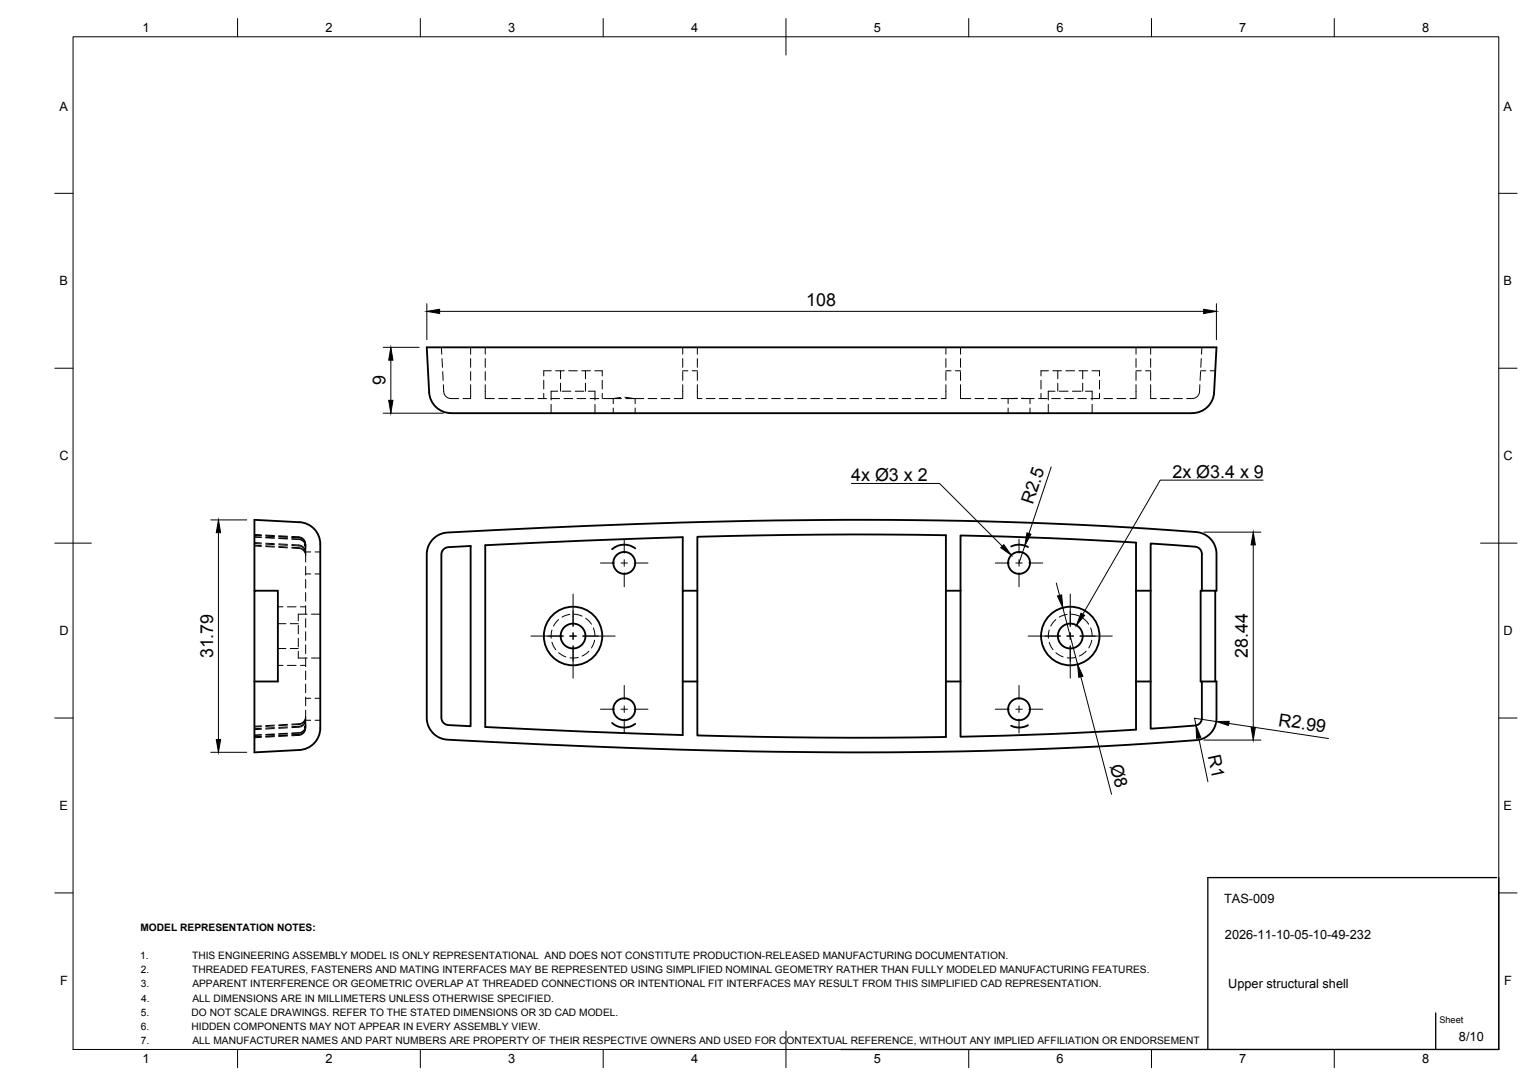
ISO-10303-21;
HEADER;
/* Generated by software containing ST-Developer
 * from STEP Tools, Inc. (www.steptools.com) 
 */

FILE_DESCRIPTION(
/* description */ (''),
/* implementation_level */ '2;1');

FILE_NAME(
/* name */ 'Upper structural shell.step',
/* time_stamp */ '2026-11-12T00:53:40-08:00',
/* author */ (''),
/* organization */ (''),
/* preprocessor_version */ 'ST-DEVELOPER v20.2',
/* originating_system */ 'Autodesk Translation Framework v15.17.0.0',
/* authorisation */ '');

FILE_SCHEMA (('AUTOMOTIVE_DESIGN { 1 0 10303 214 3 1 1 }'));
ENDSEC;

DATA;
#10=MECHANICAL_DESIGN_GEOMETRIC_PRESENTATION_REPRESENTATION('',(#575),#22129);
#76=SPHERICAL_SURFACE('',#9161,0.1);
#77=SPHERICAL_SURFACE('',#9164,0.0999999999999998);
#78=SPHERICAL_SURFACE('',#9168,0.0999999999999993);
#79=SPHERICAL_SURFACE('',#9172,0.1);
#80=SPHERICAL_SURFACE('',#9177,0.3);
#81=SPHERICAL_SURFACE('',#9181,0.3);
#82=SPHERICAL_SURFACE('',#9185,0.299999999999999);
#83=SPHERICAL_SURFACE('',#9190,0.3);
#92=B_SPLINE_SURFACE_WITH_KNOTS('',3,3,((#12365,#12366,#12367,#12368),(#12369,
#12370,#12371,#12372),(#12373,#12374,#12375,#12376),(#12377,#12378,#12379,
#12380),(#12381,#12382,#12383,#12384)),.UNSPECIFIED.,.F.,.F.,.F.,(4,1,4),
(4,4),(0.,0.571428571428571,1.),(1.0454440030657,3.44967454744645),
 .UNSPECIFIED.);
#93=B_SPLINE_SURFACE_WITH_KNOTS('',3,3,((#12457,#12458,#12459,#12460),(#12461,
#12462,#12463,#12464),(#12465,#12466,#12467,#12468),(#12469,#12470,#12471,
#12472),(#12473,#12474,#12475,#12476)),.UNSPECIFIED.,.F.,.F.,.F.,(4,1,4),
(4,4),(0.,0.571428571428571,1.),(7.24519303641511,9.95046872158573),
 .UNSPECIFIED.);
#94=B_SPLINE_SURFACE_WITH_KNOTS('',3,3,((#13338,#13339,#13340,#13341),(#13342,
#13343,#13344,#13345),(#13346,#13347,#13348,#13349),(#13350,#13351,#13352,
#13353)),.UNSPECIFIED.,.F.,.F.,.F.,(4,4),(4,4),(0.0705535719740953,0.323522444336189),
(0.0117434863834119,0.684857763552191),.UNSPECIFIED.);
#95=B_SPLINE_SURFACE_WITH_KNOTS('',3,3,((#13358,#13359,#13360,#13361),(#13362,
#13363,#13364,#13365),(#13366,#13367,#13368,#13369),(#13370,#13371,#13372,
#13373)),.UNSPECIFIED.,.F.,.F.,.F.,(4,4),(4,4),(0.0262419052680539,0.0545428296147404),
(0.0121538053864343,0.684980602226481),.UNSPECIFIED.);
#96=B_SPLINE_SURFACE_WITH_KNOTS('',3,3,((#13383,#13384,#13385,#13386),(#13387,
#13388,#13389,#13390),(#13391,#13392,#13393,#13394),(#13395,#13396,#13397,
#13398),(#13399,#13400,#13401,#13402)),.UNSPECIFIED.,.F.,.F.,.F.,(4,1,4),
(4,4),(0.,0.571428571428571,1.),(0.752061768057538,3.45733745322815),
 .UNSPECIFIED.);
#97=B_SPLINE_SURFACE_WITH_KNOTS('',3,3,((#13403,#13404,#13405,#13406),(#13407,
#13408,#13409,#13410),(#13411,#13412,#13413,#13414),(#13415,#13416,#13417,
#13418),(#13419,#13420,#13421,#13422)),.UNSPECIFIED.,.F.,.F.,.F.,(4,1,4),
(4,4),(0.,0.571428571428571,1.),(0.283259008618247,0.557056952888827),
 .UNSPECIFIED.);
#98=B_SPLINE_SURFACE_WITH_KNOTS('',3,3,((#13436,#13437,#13438,#13439),(#13440,
#13441,#13442,#13443),(#13444,#13445,#13446,#13447),(#13448,#13449,#13450,
#13451)),.UNSPECIFIED.,.F.,.F.,.F.,(4,4),(4,4),(0.67647755566375,0.929446428026011),
(0.0117434863436937,0.684857763580381),.UNSPECIFIED.);
#99=B_SPLINE_SURFACE_WITH_KNOTS('',3,3,((#13452,#13453,#13454,#13455),(#13456,
#13457,#13458,#13459),(#13460,#13461,#13462,#13463),(#13464,#13465,#13466,
#13467)),.UNSPECIFIED.,.F.,.F.,.F.,(4,4),(4,4),(0.945457170385156,0.973758094731946),
(0.0121538053598088,0.684980602226481),.UNSPECIFIED.);
#100=B_SPLINE_SURFACE_WITH_KNOTS('',3,3,((#13551,#13552,#13553,#13554),
(#13555,#13556,#13557,#13558),(#13559,#13560,#13561,#13562),(#13563,#13564,
#13565,#13566)),.UNSPECIFIED.,.F.,.F.,.F.,(4,4),(4,4),(0.341142793678372,
0.658675488550287),(0.0116221239297273,0.684255166525269),.UNSPECIFIED.);
#101=B_SPLINE_SURFACE_WITH_KNOTS('',3,3,((#13571,#13572,#13573,#13574),
(#13575,#13576,#13577,#13578),(#13579,#13580,#13581,#13582),(#13583,#13584,
#13585,#13586),(#13587,#13588,#13589,#13590)),.UNSPECIFIED.,.F.,.F.,.F.,
(4,1,4),(4,4),(0.,0.571428571428571,1.),(3.65450559744172,7.0548588409572),
 .UNSPECIFIED.);
#102=B_SPLINE_SURFACE_WITH_KNOTS('',3,3,((#13600,#13601,#13602,#13603),
(#13604,#13605,#13606,#13607),(#13608,#13609,#13610,#13611),(#13612,#13613,
#13614,#13615),(#13616,#13617,#13618,#13619)),.UNSPECIFIED.,.F.,.F.,.F.,
(4,1,4),(4,4),(0.,0.571428571428571,1.),(3.64767164868607,7.04802489220155),
 .UNSPECIFIED.);
#103=B_SPLINE_SURFACE_WITH_KNOTS('',3,3,((#13624,#13625,#13626,#13627),
(#13628,#13629,#13630,#13631),(#13632,#13633,#13634,#13635),(#13636,#13637,
#13638,#13639)),.UNSPECIFIED.,.F.,.F.,.F.,(4,4),(4,4),(0.341324511449716,
0.658857206321627),(0.0116221214776208,0.684255166525269),.UNSPECIFIED.);
#104=B_SPLINE_SURFACE_WITH_KNOTS('',3,3,((#13684,#13685,#13686,#13687),
(#13688,#13689,#13690,#13691),(#13692,#13693,#13694,#13695),(#13696,#13697,
#13698,#13699)),.UNSPECIFIED.,.F.,.F.,.F.,(4,4),(4,4),(0.676316266718331,
0.901708040522105),(0.0117102006467275,0.68495201331719),.UNSPECIFIED.);
#105=B_SPLINE_SURFACE_WITH_KNOTS('',3,3,((#13704,#13705,#13706,#13707),
(#13708,#13709,#13710,#13711),(#13712,#13713,#13714,#13715),(#13716,#13717,
#13718,#13719),(#13720,#13721,#13722,#13723)),.UNSPECIFIED.,.F.,.F.,.F.,
(4,1,4),(4,4),(0.,0.571428571428571,1.),(7.25285594219682,9.65708648657758),
 .UNSPECIFIED.);
#106=B_SPLINE_SURFACE_WITH_KNOTS('',3,3,((#13733,#13734,#13735,#13736),
(#13737,#13738,#13739,#13740),(#13741,#13742,#13743,#13744),(#13745,#13746,
#13747,#13748)),.UNSPECIFIED.,.F.,.F.,.F.,(4,4),(4,4),(0.0982919594778951,
0.323683733281714),(0.0117102006467272,0.68495201331719),.UNSPECIFIED.);
#107=B_SPLINE_SURFACE_WITH_KNOTS('',3,3,((#13823,#13824,#13825,#13826),
(#13827,#13828,#13829,#13830),(#13831,#13832,#13833,#13834),(#13835,#13836,
#13837,#13838)),.UNSPECIFIED.,.F.,.F.,.F.,(4,4),(4,4),(0.917922863855343,
0.974411608827007),(0.0122403473423911,0.685344304754238),.UNSPECIFIED.);
#108=B_SPLINE_SURFACE_WITH_KNOTS('',3,3,((#13848,#13849,#13850,#13851),
(#13852,#13853,#13854,#13855),(#13856,#13857,#13858,#13859),(#13860,#13861,
#13862,#13863),(#13864,#13865,#13866,#13867)),.UNSPECIFIED.,.F.,.F.,.F.,
(4,1,4),(4,4),(0.,0.571428571428571,1.),(9.85085636625011,10.4271318523291),
 .UNSPECIFIED.);
#109=B_SPLINE_SURFACE_WITH_KNOTS('',3,3,((#13881,#13882,#13883,#13884),
(#13885,#13886,#13887,#13888),(#13889,#13890,#13891,#13892),(#13893,#13894,
#13895,#13896)),.UNSPECIFIED.,.F.,.F.,.F.,(4,4),(4,4),(0.025588391172993,
0.0820771361446569),(0.0122403473423911,0.685344304754238),
 .UNSPECIFIED.);
#110=B_SPLINE_SURFACE_WITH_KNOTS('',3,3,((#13906,#13907,#13908,#13909),
(#13910,#13911,#13912,#13913),(#13914,#13915,#13916,#13917),(#13918,#13919,
#13920,#13921),(#13922,#13923,#13924,#13925)),.UNSPECIFIED.,.F.,.F.,.F.,
(4,1,4),(4,4),(0.,0.571428571428571,1.),(0.27539863731415,0.851674123393175),
 .UNSPECIFIED.);
#111=B_SPLINE_SURFACE_WITH_KNOTS('',3,3,((#13939,#13940,#13941,#13942),
(#13943,#13944,#13945,#13946),(#13947,#13948,#13949,#13950),(#13951,#13952,
#13953,#13954),(#13955,#13956,#13957,#13958)),.UNSPECIFIED.,.F.,.F.,.F.,
(4,1,4),(4,4),(0.,0.571428571428571,1.),(0.00944995813270487,0.618489359031386),
 .UNSPECIFIED.);
#112=B_SPLINE_SURFACE_WITH_KNOTS('',3,3,((#13965,#13966,#13967,#13968),
(#13969,#13970,#13971,#13972),(#13973,#13974,#13975,#13976),(#13977,#13978,
#13979,#13980),(#13981,#13982,#13983,#13984)),.UNSPECIFIED.,.F.,.F.,.F.,
(4,1,4),(4,4),(0.,0.571428571428571,1.),(0.00908570715245136,0.618164468641375),
 .UNSPECIFIED.);
#113=B_SPLINE_SURFACE_WITH_KNOTS('',3,3,((#13989,#13990,#13991,#13992),
(#13993,#13994,#13995,#13996),(#13997,#13998,#13999,#14000),(#14001,#14002,
#14003,#14004),(#14005,#14006,#14007,#14008)),.UNSPECIFIED.,.F.,.F.,.F.,
(4,1,4),(4,4),(0.,0.571428571428571,1.),(0.0091183540525243,0.618164468641375),
 .UNSPECIFIED.);
#114=B_SPLINE_SURFACE_WITH_KNOTS('',3,3,((#14013,#14014,#14015,#14016),
(#14017,#14018,#14019,#14020),(#14021,#14022,#14023,#14024),(#14025,#14026,
#14027,#14028),(#14029,#14030,#14031,#14032)),.UNSPECIFIED.,.F.,.F.,.F.,
(4,1,4),(4,4),(0.,0.571428571428571,1.),(10.1454735367545,10.419271481025),
 .UNSPECIFIED.);
#115=B_SPLINE_SURFACE_WITH_KNOTS('',3,3,((#14033,#14034,#14035,#14036),
(#14037,#14038,#14039,#14040),(#14041,#14042,#14043,#14044),(#14045,#14046,
#14047,#14048),(#14049,#14050,#14051,#14052)),.UNSPECIFIED.,.F.,.F.,.F.,
(4,1,4),(4,4),(0.,0.571428571428571,1.),(0.0094045468285345,0.618489359031386),
 .UNSPECIFIED.);
#116=B_SPLINE_SURFACE_WITH_KNOTS('',3,3,((#14078,#14079,#14080,#14081),
(#14082,#14083,#14084,#14085),(#14086,#14087,#14088,#14089),(#14090,#14091,
#14092,#14093),(#14094,#14095,#14096,#14097)),.UNSPECIFIED.,.F.,.F.,.F.,
(4,1,4),(4,4),(0.,0.571428571428571,1.),(-0.00535061636073277,0.618489359031386),
 .UNSPECIFIED.);
#117=B_SPLINE_SURFACE_WITH_KNOTS('',3,3,((#14116,#14117,#14118,#14119,#14120),
(#14121,#14122,#14123,#14124,#14125),(#14126,#14127,#14128,#14129,#14130),
(#14131,#14132,#14133,#14134,#14135),(#14136,#14137,#14138,#14139,#14140)),
 .UNSPECIFIED.,.F.,.F.,.F.,(4,1,4),(4,1,4),(0.,0.571428571428571,1.),(0.283259008618247,
4.63063308449434,10.4271318523291),.UNSPECIFIED.);
#118=B_SPLINE_SURFACE_WITH_KNOTS('',3,3,((#14151,#14152,#14153,#14154),
(#14155,#14156,#14157,#14158),(#14159,#14160,#14161,#14162),(#14163,#14164,
#14165,#14166),(#14167,#14168,#14169,#14170)),.UNSPECIFIED.,.F.,.F.,.F.,
(4,1,4),(4,4),(0.,0.571428571428571,1.),(-0.00578978989683084,0.618164468641375),
 .UNSPECIFIED.);
#119=B_SPLINE_SURFACE_WITH_KNOTS('',3,3,((#14179,#14180,#14181,#14182),
(#14183,#14184,#14185,#14186),(#14187,#14188,#14189,#14190),(#14191,#14192,
#14193,#14194),(#14195,#14196,#14197,#14198)),.UNSPECIFIED.,.F.,.F.,.F.,
(4,1,4),(4,4),(0.,0.571428571428571,1.),(-0.00569189159989896,0.618164468641375),
 .UNSPECIFIED.);
#120=B_SPLINE_SURFACE_WITH_KNOTS('',3,3,((#14207,#14208,#14209,#14210,#14211),
(#14212,#14213,#14214,#14215,#14216),(#14217,#14218,#14219,#14220,#14221),
(#14222,#14223,#14224,#14225,#14226),(#14227,#14228,#14229,#14230,#14231)),
 .UNSPECIFIED.,.F.,.F.,.F.,(4,1,4),(4,1,4),(0.,0.571428571428571,1.),(0.27539863731415,
4.62277271319024,10.419271481025),.UNSPECIFIED.);
#121=B_SPLINE_SURFACE_WITH_KNOTS('',3,3,((#14242,#14243,#14244,#14245),
(#14246,#14247,#14248,#14249),(#14250,#14251,#14252,#14253),(#14254,#14255,
#14256,#14257),(#14258,#14259,#14260,#14261)),.UNSPECIFIED.,.F.,.F.,.F.,
(4,1,4),(4,4),(0.,0.571428571428571,1.),(-0.0054868135546625,0.618489359031386),
 .UNSPECIFIED.);
#122=B_SPLINE_SURFACE_WITH_KNOTS('',3,3,((#14270,#14271,#14272,#14273),
(#14274,#14275,#14276,#14277),(#14278,#14279,#14280,#14281),(#14282,#14283,
#14284,#14285)),.UNSPECIFIED.,.F.,.F.,.F.,(4,4),(4,4),(0.026239262514127,
0.974414173651419),(0.,0.685344304754238),.UNSPECIFIED.);
#123=B_SPLINE_SURFACE_WITH_KNOTS('',3,3,((#14288,#14289,#14290,#14291),
(#14292,#14293,#14294,#14295),(#14296,#14297,#14298,#14299),(#14300,#14301,
#14302,#14303)),.UNSPECIFIED.,.F.,.F.,.F.,(4,4),(4,4),(0.0255858263485814,
0.973760737485873),(0.,0.685344304754238),.UNSPECIFIED.);
#172=B_SPLINE_CURVE_WITH_KNOTS('',3,(#12264,#12265,#12266,#12267,#12268,
#12269,#12270,#12271,#12272,#12273,#12274,#12275,#12276,#12277,#12278,#12279,
#12280,#12281,#12282,#12283,#12284,#12285,#12286,#12287),.UNSPECIFIED.,
 .F.,.F.,(4,2,2,2,2,2,2,2,2,2,2,4),(-0.337265338267783,-0.250544943628509,
-0.208272806508042,-0.186542211788094,-0.176382978682897,-0.170925844043069,
-0.16639450677335,-0.161077381235501,-0.15182241135393,-0.115009181549223,
-0.030206004227969,0.),.UNSPECIFIED.);
#173=B_SPLINE_CURVE_WITH_KNOTS('',3,(#12292,#12293,#12294,#12295,#12296,
#12297,#12298,#12299,#12300,#12301,#12302,#12303,#12304,#12305,#12306,#12307,
#12308,#12309,#12310,#12311),.UNSPECIFIED.,.F.,.F.,(4,2,2,2,2,2,2,2,2,4),
(-0.240982594686416,-0.16829976149504,-0.141836598208813,-0.129116059226128,
-0.121962912034391,-0.115857591426886,-0.108506552485159,-0.0948769875819265,
-0.0364654790774683,0.),.UNSPECIFIED.);
#174=B_SPLINE_CURVE_WITH_KNOTS('',3,(#12316,#12317,#12318,#12319,#12320,
#12321,#12322,#12323,#12324,#12325,#12326,#12327,#12328,#12329,#12330,#12331,
#12332,#12333,#12334,#12335),.UNSPECIFIED.,.F.,.F.,(4,2,2,2,2,2,2,2,2,4),
(-0.240981214998207,-0.168303541671295,-0.141841407502325,-0.129121097580905,
-0.121968013294536,-0.115862708924237,-0.108511643765797,-0.0948818976588229,
-0.0364681276985956,0.),.UNSPECIFIED.);
#175=B_SPLINE_CURVE_WITH_KNOTS('',3,(#12340,#12341,#12342,#12343,#12344,
#12345,#12346,#12347,#12348,#12349,#12350,#12351,#12352,#12353,#12354,#12355,
#12356,#12357,#12358,#12359,#12360,#12361,#12362,#12363),.UNSPECIFIED.,
 .F.,.F.,(4,2,2,2,2,2,2,2,2,2,2,4),(-0.337269388373684,-0.250545316912909,
-0.208282401844766,-0.186554569827561,-0.176396213396297,-0.17093921790305,
-0.16640782243471,-0.161090427650893,-0.151834477986603,-0.115010808423941,
-0.0302102096065556,0.),.UNSPECIFIED.);
#176=B_SPLINE_CURVE_WITH_KNOTS('',3,(#12386,#12387,#12388,#12389),
 .UNSPECIFIED.,.F.,.F.,(4,4),(1.0454440030657,2.52465537163019),
 .UNSPECIFIED.);
#177=B_SPLINE_CURVE_WITH_KNOTS('',3,(#12391,#12392,#12393,#12394,#12395,
#12396,#12397,#12398,#12399,#12400,#12401,#12402,#12403,#12404,#12405,#12406,
#12407,#12408,#12409,#12410,#12411,#12412,#12413,#12414,#12415,#12416,#12417,
#12418),.UNSPECIFIED.,.F.,.F.,(4,3,3,3,3,3,3,3,3,4),(-0.152193408756968,
-0.128427023368412,-0.115107736263918,-0.0911810900745799,-0.0780377802127556,
-0.0652031397886901,-0.0414031558437525,-0.0389949527774582,-0.0152076153333754,
0.),.UNSPECIFIED.);
#178=B_SPLINE_CURVE_WITH_KNOTS('',3,(#12420,#12421,#12422,#12423),
 .UNSPECIFIED.,.F.,.F.,(4,4),(-3.44967454744645,-1.05170160817356),
 .UNSPECIFIED.);
#179=B_SPLINE_CURVE_WITH_KNOTS('',3,(#12425,#12426,#12427,#12428,#12429,
#12430,#12431,#12432,#12433,#12434,#12435,#12436,#12437,#12438,#12439,#12440,
#12441,#12442,#12443,#12444,#12445,#12446,#12447,#12448,#12449,#12450,#12451,
#12452),.UNSPECIFIED.,.F.,.F.,(4,3,3,3,3,3,3,3,3,4),(-0.152278960443096,
-0.128503570101575,-0.115218572146868,-0.09145408274965,-0.0870214650669139,
-0.0781562978024333,-0.0542566895399357,-0.03908030849237,-0.0153296112319379,
0.),.UNSPECIFIED.);
#180=B_SPLINE_CURVE_WITH_KNOTS('',3,(#12453,#12454,#12455,#12456),
 .UNSPECIFIED.,.F.,.F.,(4,4),(2.75501813708031,3.4476340663212),
 .UNSPECIFIED.);
#181=B_SPLINE_CURVE_WITH_KNOTS('',3,(#12478,#12479,#12480,#12481),
 .UNSPECIFIED.,.F.,.F.,(4,4),(7.24810383506675,7.89761558728778),
 .UNSPECIFIED.);
#182=B_SPLINE_CURVE_WITH_KNOTS('',3,(#12483,#12484,#12485,#12486,#12487,
#12488,#12489,#12490,#12491,#12492,#12493,#12494,#12495,#12496,#12497,#12498,
#12499,#12500,#12501,#12502,#12503,#12504,#12505,#12506,#12507,#12508,#12509,
#12510),.UNSPECIFIED.,.F.,.F.,(4,3,3,3,3,3,3,3,3,4),(-0.152278869104567,
-0.128548794904564,-0.115192257893812,-0.0912773536606376,-0.0781090575823055,
-0.0652724057916263,-0.0414819581560496,-0.0390493575290778,-0.015259721743698,
0.),.UNSPECIFIED.);
#183=B_SPLINE_CURVE_WITH_KNOTS('',3,(#12512,#12513,#12514,#12515),
 .UNSPECIFIED.,.F.,.F.,(4,4),(-9.94532343034734,-7.24519303641511),
 .UNSPECIFIED.);
#184=B_SPLINE_CURVE_WITH_KNOTS('',3,(#12517,#12518,#12519,#12520,#12521,
#12522,#12523,#12524,#12525,#12526,#12527,#12528,#12529,#12530,#12531,#12532,
#12533,#12534,#12535,#12536,#12537,#12538,#12539,#12540,#12541,#12542,#12543,
#12544),.UNSPECIFIED.,.F.,.F.,(4,3,3,3,3,3,3,3,3,4),(-0.152181623618259,
-0.128410404494075,-0.115248188224843,-0.0914746846046984,-0.0869904866333268,
-0.0783028696190655,-0.0543945376065823,-0.0391651209697638,-0.0153884182770307,
0.),.UNSPECIFIED.);
#185=B_SPLINE_CURVE_WITH_KNOTS('',3,(#12545,#12546,#12547,#12548),
 .UNSPECIFIED.,.F.,.F.,(4,4),(8.21380824320284,9.95046871680089),
 .UNSPECIFIED.);
#186=B_SPLINE_CURVE_WITH_KNOTS('',3,(#12551,#12552,#12553,#12554),
 .UNSPECIFIED.,.F.,.F.,(4,4),(2.80491490332713,3.45442665446657),
 .UNSPECIFIED.);
#187=B_SPLINE_CURVE_WITH_KNOTS('',3,(#12558,#12559,#12560,#12561),
 .UNSPECIFIED.,.F.,.F.,(4,4),(0.752061768057538,2.48872224644044),
 .UNSPECIFIED.);
#188=B_SPLINE_CURVE_WITH_KNOTS('',3,(#12709,#12710,#12711,#12712,#12713,
#12714),.UNSPECIFIED.,.F.,.F.,(4,2,4),(-0.606700505977711,-0.303383635264422,
-0.000339350725729326),.UNSPECIFIED.);
#189=B_SPLINE_CURVE_WITH_KNOTS('',3,(#12715,#12716,#12717,#12718,#12719,
#12720,#12721,#12722,#12723,#12724,#12725,#12726,#12727,#12728,#12729,#12730,
#12731,#12732,#12733,#12734,#12735,#12736,#12737,#12738,#12739,#12740,#12741,
#12742),.UNSPECIFIED.,.F.,.F.,(4,3,3,3,3,3,3,3,3,4),(-0.152173579228948,
-0.128423230539522,-0.115115104157663,-0.0911927259648815,-0.0780672068328041,
-0.0652082609452843,-0.0414117413801899,-0.0390174000215468,-0.0152300060615686,
0.),.UNSPECIFIED.);
#190=B_SPLINE_CURVE_WITH_KNOTS('',3,(#12743,#12744,#12745,#12746,#12747,
#12748),.UNSPECIFIED.,.F.,.F.,(4,2,4),(-0.606471894652381,-0.303383500305553,
-0.00011071898471493),.UNSPECIFIED.);
#191=B_SPLINE_CURVE_WITH_KNOTS('',3,(#12752,#12753,#12754,#12755,#12756,
#12757),.UNSPECIFIED.,.F.,.F.,(4,2,4),(-0.606240625011114,-0.303433113375332,
-0.00010938105916114),.UNSPECIFIED.);
#192=B_SPLINE_CURVE_WITH_KNOTS('',3,(#12759,#12760,#12761,#12762,#12763,
#12764,#12765,#12766,#12767,#12768,#12769,#12770,#12771,#12772,#12773,#12774,
#12775,#12776,#12777,#12778,#12779,#12780,#12781,#12782,#12783,#12784,#12785,
#12786),.UNSPECIFIED.,.F.,.F.,(4,3,3,3,3,3,3,3,3,4),(-0.152281454644235,
-0.128508102092242,-0.115234945630277,-0.0914677943501604,-0.0870276017853555,
-0.0781846052914712,-0.0542821334115454,-0.0390966859411886,-0.0153419673568312,
0.),.UNSPECIFIED.);
#193=B_SPLINE_CURVE_WITH_KNOTS('',3,(#12788,#12789,#12790,#12791,#12792,
#12793),.UNSPECIFIED.,.F.,.F.,(4,2,4),(-0.606758573154242,-0.303433157101101,
-0.000627306481538803),.UNSPECIFIED.);
#194=B_SPLINE_CURVE_WITH_KNOTS('',3,(#12799,#12800,#12801,#12802,#12803,
#12804),.UNSPECIFIED.,.F.,.F.,(4,2,4),(-0.60617382748,-0.303436117212405,
-7.2700296824213E-5),.UNSPECIFIED.);
#195=B_SPLINE_CURVE_WITH_KNOTS('',3,(#12806,#12807,#12808,#12809,#12810,
#12811,#12812,#12813,#12814,#12815,#12816,#12817,#12818,#12819,#12820,#12821,
#12822,#12823,#12824,#12825,#12826,#12827,#12828,#12829,#12830,#12831,#12832,
#12833),.UNSPECIFIED.,.F.,.F.,(4,3,3,3,3,3,3,3,3,4),(-0.152282154327755,
-0.128558036203745,-0.115201429639692,-0.0912891813973639,-0.0781219052297615,
-0.065279687589213,-0.0414913146723999,-0.0390591331507366,-0.0152683745546824,
0.),.UNSPECIFIED.);
#196=B_SPLINE_CURVE_WITH_KNOTS('',3,(#12837,#12838,#12839,#12840,#12841,
#12842,#12843,#12844,#12845,#12846,#12847,#12848,#12849,#12850,#12851,#12852,
#12853,#12854,#12855,#12856,#12857,#12858,#12859,#12860,#12861,#12862,#12863,
#12864),.UNSPECIFIED.,.F.,.F.,(4,3,3,3,3,3,3,3,3,4),(-0.152283066055976,
-0.128508717930245,-0.115216472798554,-0.091451700383826,-0.087022506454752,
-0.0781485278686168,-0.0542483994686567,-0.0390758108455304,-0.0153274175274101,
0.),.UNSPECIFIED.);
#197=B_SPLINE_CURVE_WITH_KNOTS('',3,(#12866,#12867,#12868,#12869,#12870,
#12871),.UNSPECIFIED.,.F.,.F.,(4,2,4),(-0.606800264911061,-0.303436147592132,
-0.000699137727853738),.UNSPECIFIED.);
#198=B_SPLINE_CURVE_WITH_KNOTS('',3,(#12876,#12877,#12878,#12879,#12880,
#12881),.UNSPECIFIED.,.F.,.F.,(4,2,4),(-0.606915279655722,-0.30363236403835,
-0.000516487074480598),.UNSPECIFIED.);
#199=B_SPLINE_CURVE_WITH_KNOTS('',3,(#12885,#12886,#12887,#12888,#12889,
#12890,#12891,#12892,#12893,#12894,#12895,#12896,#12897,#12898,#12899,#12900,
#12901,#12902,#12903,#12904,#12905,#12906,#12907,#12908,#12909,#12910,#12911,
#12912),.UNSPECIFIED.,.F.,.F.,(4,3,3,3,3,3,3,3,3,4),(-0.152205325335401,
-0.128433618138404,-0.115304790388008,-0.091527299141506,-0.0870178586418932,
-0.0783866443643876,-0.0544751548276533,-0.0392137310602028,-0.0154203878854647,
0.),.UNSPECIFIED.);
#200=B_SPLINE_CURVE_WITH_KNOTS('',3,(#12914,#12915,#12916,#12917,#12918,
#12919),.UNSPECIFIED.,.F.,.F.,(4,2,4),(-0.606752424187958,-0.303632696349781,
-0.000353591088346872),.UNSPECIFIED.);
#201=B_SPLINE_CURVE_WITH_KNOTS('',3,(#12925,#12926,#12927,#12928),
 .UNSPECIFIED.,.F.,.F.,(4,4),(0.0116023361771303,0.618489359031386),
 .UNSPECIFIED.);
#202=B_SPLINE_CURVE_WITH_KNOTS('',3,(#12932,#12933,#12934,#12935),
 .UNSPECIFIED.,.F.,.F.,(4,4),(-0.618489359031386,-0.01160233617713),
 .UNSPECIFIED.);
#203=B_SPLINE_CURVE_WITH_KNOTS('',3,(#12938,#12939,#12940,#12941),
 .UNSPECIFIED.,.F.,.F.,(4,4),(7.01593971618694,9.71770560667459),
 .UNSPECIFIED.);
#204=B_SPLINE_CURVE_WITH_KNOTS('',3,(#12942,#12943,#12944,#12945),
 .UNSPECIFIED.,.F.,.F.,(4,4),(0.505945342046796,3.20718651982575),
 .UNSPECIFIED.);
#205=B_SPLINE_CURVE_WITH_KNOTS('',3,(#12948,#12949,#12950,#12951,#12952,
#12953,#12954),.UNSPECIFIED.,.F.,.F.,(4,3,4),(3.40717417387402,5.11170895874517,
6.80746068626633),.UNSPECIFIED.);
#206=B_SPLINE_CURVE_WITH_KNOTS('',3,(#12957,#12958,#12959,#12960),
 .UNSPECIFIED.,.F.,.F.,(4,4),(7.00766573366377,9.41198845520559),
 .UNSPECIFIED.);
#207=B_SPLINE_CURVE_WITH_KNOTS('',3,(#12964,#12965,#12966,#12967),
 .UNSPECIFIED.,.F.,.F.,(4,4),(9.61248784142317,10.2217363065808),
 .UNSPECIFIED.);
#208=B_SPLINE_CURVE_WITH_KNOTS('',3,(#12968,#12969,#12970,#12971,#12972,
#12973,#12974,#12975,#12976,#12977,#12978,#12979,#12980,#12981,#12982,#12983,
#12984,#12985,#12986,#12987,#12988,#12989,#12990,#12991,#12992,#12993,#12994,
#12995),.UNSPECIFIED.,.F.,.F.,(4,3,3,3,3,3,3,3,3,4),(0.,0.0238103109064959,
0.0390781362249314,0.0628635086275546,0.0641230352384255,0.0780643700703951,
0.101962174814111,0.113803522271848,0.137549611554782,0.149564734365165),
 .UNSPECIFIED.);
#209=B_SPLINE_CURVE_WITH_KNOTS('',3,(#12999,#13000,#13001,#13002,#13003,
#13004,#13005,#13006,#13007,#13008,#13009,#13010,#13011,#13012,#13013,#13014,
#13015,#13016,#13017,#13018,#13019,#13020,#13021,#13022,#13023,#13024,#13025,
#13026,#13027,#13028,#13029),.UNSPECIFIED.,.F.,.F.,(4,3,3,3,3,3,3,3,3,3,
4),(0.,0.0535521515156599,0.107729685495911,0.117233338918226,0.171447998942947,
0.1923696899792,0.234191611538245,0.288659693466396,0.341410301570312,0.395549383747909,
0.448696573746633),.UNSPECIFIED.);
#210=B_SPLINE_CURVE_WITH_KNOTS('',3,(#13031,#13032,#13033,#13034),
 .UNSPECIFIED.,.F.,.F.,(4,4),(0.0255858263485814,0.973760737485873),
 .UNSPECIFIED.);
#211=B_SPLINE_CURVE_WITH_KNOTS('',3,(#13036,#13037,#13038,#13039,#13040,
#13041,#13042,#13043,#13044,#13045,#13046,#13047,#13048,#13049,#13050,#13051,
#13052,#13053,#13054,#13055,#13056,#13057,#13058,#13059,#13060,#13061,#13062,
#13063,#13064,#13065,#13066),.UNSPECIFIED.,.F.,.F.,(4,3,3,3,3,3,3,3,3,3,
4),(0.,0.0535144560117858,0.107726856902975,0.117300577410231,0.171517675930231,
0.195438847090422,0.234297456941738,0.289665153342662,0.345032849743585,
0.40043206955427,0.455831289364955),.UNSPECIFIED.);
#212=B_SPLINE_CURVE_WITH_KNOTS('',3,(#13070,#13071,#13072,#13073,#13074,
#13075,#13076,#13077,#13078,#13079,#13080,#13081,#13082,#13083,#13084,#13085,
#13086,#13087,#13088,#13089,#13090,#13091,#13092,#13093,#13094,#13095,#13096,
#13097,#13098,#13099,#13100),.UNSPECIFIED.,.F.,.F.,(4,3,3,3,3,3,3,3,3,3,
4),(0.,0.053505543180391,0.107714168832353,0.117253997025819,0.171473395203321,
0.195418854185489,0.234223199196375,0.289607016015183,0.344990832833991,
0.400409777473312,0.455828722112633),.UNSPECIFIED.);
#213=B_SPLINE_CURVE_WITH_KNOTS('',3,(#13102,#13103,#13104,#13105),
 .UNSPECIFIED.,.F.,.F.,(4,4),(0.0262392625141271,0.974414173651419),
 .UNSPECIFIED.);
#214=B_SPLINE_CURVE_WITH_KNOTS('',3,(#13107,#13108,#13109,#13110,#13111,
#13112,#13113,#13114,#13115,#13116,#13117,#13118,#13119,#13120,#13121,#13122,
#13123,#13124,#13125,#13126,#13127,#13128,#13129,#13130,#13131,#13132,#13133,
#13134,#13135,#13136,#13137),.UNSPECIFIED.,.F.,.F.,(4,3,3,3,3,3,3,3,3,3,
4),(0.,0.0535648734523888,0.107747221190676,0.117299947751206,0.171510987106922,
0.192397607227928,0.234296687348373,0.288768001369001,0.341469499352622,
0.395597672314973,0.448700135162036),.UNSPECIFIED.);
#215=B_SPLINE_CURVE_WITH_KNOTS('',3,(#13140,#13141,#13142,#13143,#13144,
#13145,#13146,#13147,#13148,#13149,#13150,#13151,#13152,#13153,#13154,#13155,
#13156,#13157,#13158,#13159,#13160,#13161,#13162,#13163,#13164),
 .UNSPECIFIED.,.F.,.F.,(4,3,3,3,3,3,3,3,4),(0.,0.0238141989470671,0.0391004231578824,
0.0641320992313133,0.0780996136084711,0.101998806889826,0.113823260594808,
0.137564745199532,0.149565921982294),.UNSPECIFIED.);
#216=B_SPLINE_CURVE_WITH_KNOTS('',3,(#13166,#13167,#13168,#13169),
 .UNSPECIFIED.,.F.,.F.,(4,4),(2.76692059912875E-5,0.609394470571143),
 .UNSPECIFIED.);
#217=B_SPLINE_CURVE_WITH_KNOTS('',3,(#13172,#13173,#13174,#13175),
 .UNSPECIFIED.,.F.,.F.,(4,4),(0.809932799154201,3.21472245120952),
 .UNSPECIFIED.);
#218=B_SPLINE_CURVE_WITH_KNOTS('',3,(#13178,#13179,#13180,#13181,#13182,
#13183,#13184),.UNSPECIFIED.,.F.,.F.,(4,3,4),(3.41496637450242,5.11093193409745,
6.81591321610411),.UNSPECIFIED.);
#219=B_SPLINE_CURVE_WITH_KNOTS('',3,(#13188,#13189,#13190,#13191),
 .UNSPECIFIED.,.F.,.F.,(4,4),(9.91798263530139,10.2237206759544),
 .UNSPECIFIED.);
#220=B_SPLINE_CURVE_WITH_KNOTS('',3,(#13193,#13194,#13195,#13196,#13197,
#13198,#13199,#13200,#13201,#13202,#13203,#13204,#13205,#13206,#13207,#13208,
#13209,#13210,#13211,#13212,#13213,#13214,#13215,#13216,#13217,#13218,#13219,
#13220),.UNSPECIFIED.,.F.,.F.,(4,3,3,3,3,3,3,3,3,4),(0.,0.023807020713713,
0.039085080816122,0.0628703378723092,0.0651394887354207,0.0780750047750988,
0.101981498769656,0.114997221725907,0.138748569029605,0.151942344104828),
 .UNSPECIFIED.);
#221=B_SPLINE_CURVE_WITH_KNOTS('',3,(#13224,#13225,#13226,#13227,#13228,
#13229,#13230,#13231,#13232,#13233,#13234,#13235,#13236,#13237,#13238,#13239,
#13240,#13241,#13242,#13243,#13244,#13245,#13246,#13247,#13248,#13249,#13250,
#13251),.UNSPECIFIED.,.F.,.F.,(4,3,3,3,3,3,3,3,3,4),(0.,0.0238098191818892,
0.0391006681981376,0.0628849269680955,0.0651459659463291,0.0780999162396042,
0.102007524384594,0.115011225379555,0.138759376430353,0.151943200125079),
 .UNSPECIFIED.);
#222=B_SPLINE_CURVE_WITH_KNOTS('',3,(#13253,#13254,#13255,#13256),
 .UNSPECIFIED.,.F.,.F.,(4,4),(2.85486020485948E-5,0.305707210239178),
 .UNSPECIFIED.);
#223=B_SPLINE_CURVE_WITH_KNOTS('',3,(#13266,#13267,#13268,#13269,#13270,
#13271),.UNSPECIFIED.,.F.,.F.,(4,2,4),(-0.606446248197249,-0.303383959626182,
-6.4365448350312E-5),.UNSPECIFIED.);
#224=B_SPLINE_CURVE_WITH_KNOTS('',3,(#13273,#13274,#13275,#13276,#13277,
#13278),.UNSPECIFIED.,.F.,.F.,(4,2,4),(-0.60675170080159,-0.303384112192838,
-0.000369837888147484),.UNSPECIFIED.);
#225=B_SPLINE_CURVE_WITH_KNOTS('',3,(#13280,#13281,#13282,#13283,#13284,
#13285,#13286,#13287,#13288,#13289,#13290,#13291,#13292,#13293,#13294,#13295,
#13296,#13297,#13298,#13299,#13300,#13301,#13302,#13303,#13304,#13305,#13306,
#13307),.UNSPECIFIED.,.F.,.F.,(4,3,3,3,3,3,3,3,3,4),(-0.152162866344201,
-0.128411131698784,-0.115108013904405,-0.0911850729173883,-0.0780642464630149,
-0.0652023242402653,-0.0414053499882389,-0.0390151293250392,-0.0152279490549848,
0.),.UNSPECIFIED.);
#226=B_SPLINE_CURVE_WITH_KNOTS('',3,(#13310,#13311,#13312,#13313,#13314,
#13315,#13316,#13317,#13318,#13319,#13320,#13321,#13322,#13323,#13324,#13325,
#13326,#13327,#13328,#13329,#13330,#13331,#13332,#13333,#13334,#13335,#13336,
#13337),.UNSPECIFIED.,.F.,.F.,(4,3,3,3,3,3,3,3,3,4),(-0.152171297476962,
-0.128400300768352,-0.115247520946962,-0.0914735511738372,-0.0869860114952295,
-0.0783112904282795,-0.0544025203706761,-0.0391699941254272,-0.015391764586027,
0.),.UNSPECIFIED.);
#227=B_SPLINE_CURVE_WITH_KNOTS('',3,(#13354,#13355,#13356,#13357),
 .UNSPECIFIED.,.F.,.F.,(4,4),(-3.45733745322815,-0.757207059295936),
 .UNSPECIFIED.);
#228=B_SPLINE_CURVE_WITH_KNOTS('',3,(#13375,#13376,#13377,#13378),
 .UNSPECIFIED.,.F.,.F.,(4,4),(-0.557056952888827,-0.283259008618247),
 .UNSPECIFIED.);
#229=B_SPLINE_CURVE_WITH_KNOTS('',3,(#13379,#13380,#13381,#13382),
 .UNSPECIFIED.,.F.,.F.,(4,4),(-0.618164468641375,-0.0110156167597059),
 .UNSPECIFIED.);
#230=B_SPLINE_CURVE_WITH_KNOTS('',3,(#13424,#13425,#13426,#13427),
 .UNSPECIFIED.,.F.,.F.,(4,4),(0.283259011433088,0.551788488929761),
 .UNSPECIFIED.);
#231=B_SPLINE_CURVE_WITH_KNOTS('',3,(#13431,#13432,#13433,#13434),
 .UNSPECIFIED.,.F.,.F.,(4,4),(10.1507419987596,10.419271481025),
 .UNSPECIFIED.);
#232=B_SPLINE_CURVE_WITH_KNOTS('',3,(#13469,#13470,#13471,#13472),
 .UNSPECIFIED.,.F.,.F.,(4,4),(0.0110156167597055,0.618164468641375),
 .UNSPECIFIED.);
#233=B_SPLINE_CURVE_WITH_KNOTS('',3,(#13473,#13474,#13475,#13476),
 .UNSPECIFIED.,.F.,.F.,(4,4),(-10.419271481025,-10.1454735367545),
 .UNSPECIFIED.);
#234=B_SPLINE_CURVE_WITH_KNOTS('',3,(#13479,#13480,#13481,#13482,#13483,
#13484),.UNSPECIFIED.,.F.,.F.,(4,2,4),(-0.606211482799139,-0.303431960476852,
-9.19895310989571E-5),.UNSPECIFIED.);
#235=B_SPLINE_CURVE_WITH_KNOTS('',3,(#13486,#13487,#13488,#13489,#13490,
#13491,#13492,#13493,#13494,#13495,#13496,#13497,#13498,#13499,#13500,#13501,
#13502,#13503,#13504,#13505,#13506,#13507,#13508,#13509,#13510,#13511,#13512,
#13513),.UNSPECIFIED.,.F.,.F.,(4,3,3,3,3,3,3,3,3,4),(-0.152283340966725,
-0.128554242174982,-0.115196092098682,-0.0912819860997417,-0.0781117853096875,
-0.0652755629514801,-0.0414857317972147,-0.039051434275634,-0.0152612146291672,
0.),.UNSPECIFIED.);
#236=B_SPLINE_CURVE_WITH_KNOTS('',3,(#13517,#13518,#13519,#13520,#13521,
#13522,#13523,#13524,#13525,#13526,#13527,#13528,#13529,#13530,#13531,#13532,
#13533,#13534,#13535,#13536,#13537,#13538,#13539,#13540,#13541,#13542,#13543,
#13544),.UNSPECIFIED.,.F.,.F.,(4,3,3,3,3,3,3,3,3,4),(-0.152285570909379,
-0.128511627155755,-0.115232904621082,-0.0914664612111958,-0.0870286654075453,
-0.0781769338106538,-0.0542752301960614,-0.039092246575741,-0.0153386136911565,
0.),.UNSPECIFIED.);
#237=B_SPLINE_CURVE_WITH_KNOTS('',3,(#13545,#13546,#13547,#13548,#13549,
#13550),.UNSPECIFIED.,.F.,.F.,(4,2,4),(-0.606773318344362,-0.303431998667662,
-0.000653802131222458),.UNSPECIFIED.);
#238=B_SPLINE_CURVE_WITH_KNOTS('',3,(#13567,#13568,#13569,#13570),
 .UNSPECIFIED.,.F.,.F.,(4,4),(-7.05313168653828,-3.6572084986735),
 .UNSPECIFIED.);
#239=B_SPLINE_CURVE_WITH_KNOTS('',3,(#13591,#13592,#13593,#13594),
 .UNSPECIFIED.,.F.,.F.,(4,4),(3.65450559744172,7.0548588409572),
 .UNSPECIFIED.);
#240=B_SPLINE_CURVE_WITH_KNOTS('',3,(#13596,#13597,#13598,#13599),
 .UNSPECIFIED.,.F.,.F.,(4,4),(3.64767164868607,7.04802489220155),
 .UNSPECIFIED.);
#241=B_SPLINE_CURVE_WITH_KNOTS('',3,(#13620,#13621,#13622,#13623),
 .UNSPECIFIED.,.F.,.F.,(4,4),(-7.04532199096977,-3.64939880310499),
 .UNSPECIFIED.);
#242=B_SPLINE_CURVE_WITH_KNOTS('',3,(#13642,#13643,#13644,#13645,#13646,
#13647),.UNSPECIFIED.,.F.,.F.,(4,2,4),(-0.606200453641641,-0.30343602424441,
-9.0120313562092E-5),.UNSPECIFIED.);
#243=B_SPLINE_CURVE_WITH_KNOTS('',3,(#13649,#13650,#13651,#13652,#13653,
#13654,#13655,#13656,#13657,#13658,#13659,#13660,#13661,#13662,#13663,#13664,
#13665,#13666,#13667,#13668,#13669,#13670,#13671,#13672,#13673,#13674,#13675,
#13676),.UNSPECIFIED.,.F.,.F.,(4,3,3,3,3,3,3,3,3,4),(-0.152277688086818,
-0.128551334178815,-0.115197577176818,-0.0912856014461669,-0.0781191417238373,
-0.0652765169533013,-0.0414883027365163,-0.0390570310290822,-0.0152653090895913,
0.),.UNSPECIFIED.);
#244=B_SPLINE_CURVE_WITH_KNOTS('',3,(#13678,#13679,#13680,#13681,#13682,
#13683),.UNSPECIFIED.,.F.,.F.,(4,2,4),(-0.60678286609787,-0.303436074842897,
-0.000672492961417026),.UNSPECIFIED.);
#245=B_SPLINE_CURVE_WITH_KNOTS('',3,(#13700,#13701,#13702,#13703),
 .UNSPECIFIED.,.F.,.F.,(4,4),(-9.65082888146972,-7.25285594219682),
 .UNSPECIFIED.);
#246=B_SPLINE_CURVE_WITH_KNOTS('',3,(#13724,#13725,#13726,#13727),
 .UNSPECIFIED.,.F.,.F.,(4,4),(7.25489642332205,7.94751235889625),
 .UNSPECIFIED.);
#247=B_SPLINE_CURVE_WITH_KNOTS('',3,(#13728,#13729,#13730,#13731),
 .UNSPECIFIED.,.F.,.F.,(4,4),(8.17787511801303,9.65708648657758),
 .UNSPECIFIED.);
#248=B_SPLINE_CURVE_WITH_KNOTS('',3,(#13751,#13752,#13753,#13754,#13755,
#13756),.UNSPECIFIED.,.F.,.F.,(4,2,4),(-0.607007797795788,-0.303636495504298,
-0.000571323176327465),.UNSPECIFIED.);
#249=B_SPLINE_CURVE_WITH_KNOTS('',3,(#13758,#13759,#13760,#13761,#13762,
#13763,#13764,#13765,#13766,#13767,#13768,#13769,#13770,#13771,#13772,#13773,
#13774,#13775,#13776,#13777,#13778,#13779,#13780,#13781,#13782,#13783,#13784,
#13785),.UNSPECIFIED.,.F.,.F.,(4,3,3,3,3,3,3,3,3,4),(-0.152184339020145,
-0.128410461444444,-0.115096394428865,-0.0911692948751363,-0.0780261759644403,
-0.0651939085034322,-0.0413932235702045,-0.0389860720679279,-0.0151971168406065,
0.),.UNSPECIFIED.);
#250=B_SPLINE_CURVE_WITH_KNOTS('',3,(#13789,#13790,#13791,#13792,#13793,
#13794,#13795,#13796,#13797,#13798,#13799,#13800,#13801,#13802,#13803,#13804,
#13805,#13806,#13807,#13808,#13809,#13810,#13811,#13812,#13813,#13814,#13815,
#13816),.UNSPECIFIED.,.F.,.F.,(4,3,3,3,3,3,3,3,3,4),(-0.15219777746951,
-0.128424216118147,-0.115318679085322,-0.0915406112613293,-0.0870190514838729,
-0.0784197287877601,-0.0545085386658457,-0.0392329067084975,-0.0154317870320417,
0.),.UNSPECIFIED.);
#251=B_SPLINE_CURVE_WITH_KNOTS('',3,(#13817,#13818,#13819,#13820,#13821,
#13822),.UNSPECIFIED.,.F.,.F.,(4,2,4),(-0.606706256981509,-0.303636876939173,
-0.00026974181288697),.UNSPECIFIED.);
#252=B_SPLINE_CURVE_WITH_KNOTS('',3,(#13840,#13841,#13842,#13843),
 .UNSPECIFIED.,.F.,.F.,(4,4),(0.0112334529114386,0.618489359031386),
 .UNSPECIFIED.);
#253=B_SPLINE_CURVE_WITH_KNOTS('',3,(#13844,#13845,#13846,#13847),
 .UNSPECIFIED.,.F.,.F.,(4,4),(-10.4271318523291,-9.85085636625011),
 .UNSPECIFIED.);
#254=B_SPLINE_CURVE_WITH_KNOTS('',3,(#13870,#13871,#13872,#13873),
 .UNSPECIFIED.,.F.,.F.,(4,4),(9.85750350611301,10.4271318523291),
 .UNSPECIFIED.);
#255=B_SPLINE_CURVE_WITH_KNOTS('',3,(#13877,#13878,#13879,#13880),
 .UNSPECIFIED.,.F.,.F.,(4,4),(0.27539863731415,0.845026983530265),
 .UNSPECIFIED.);
#256=B_SPLINE_CURVE_WITH_KNOTS('',3,(#13898,#13899,#13900,#13901),
 .UNSPECIFIED.,.F.,.F.,(4,4),(-0.851674123393175,-0.27539863731415),
 .UNSPECIFIED.);
#257=B_SPLINE_CURVE_WITH_KNOTS('',3,(#13902,#13903,#13904,#13905),
 .UNSPECIFIED.,.F.,.F.,(4,4),(-0.618489359031386,-0.0112334529114389),
 .UNSPECIFIED.);
#258=B_SPLINE_CURVE_WITH_KNOTS('',3,(#13985,#13986,#13987,#13988),
 .UNSPECIFIED.,.F.,.F.,(4,4),(0.0112755522169305,0.618164468641375),
 .UNSPECIFIED.);
#259=B_SPLINE_CURVE_WITH_KNOTS('',3,(#14009,#14010,#14011,#14012),
 .UNSPECIFIED.,.F.,.F.,(4,4),(-0.618164468641375,-0.0112755522169305),
 .UNSPECIFIED.);
#260=B_SPLINE_CURVE_WITH_KNOTS('',3,(#14098,#14099,#14100,#14101),
 .UNSPECIFIED.,.F.,.F.,(4,4),(5.55111512312578E-17,0.618489359031386),
 .UNSPECIFIED.);
#261=B_SPLINE_CURVE_WITH_KNOTS('',3,(#14102,#14103,#14104,#14105),
 .UNSPECIFIED.,.F.,.F.,(4,4),(-0.618489359031386,-0.00110654915602034),
 .UNSPECIFIED.);
#262=B_SPLINE_CURVE_WITH_KNOTS('',3,(#14141,#14142,#14143,#14144,#14145),
 .UNSPECIFIED.,.F.,.F.,(4,1,4),(-10.4271318523291,-4.63063308449434,-0.283259008618247),
 .UNSPECIFIED.);
#263=B_SPLINE_CURVE_WITH_KNOTS('',3,(#14146,#14147,#14148,#14149,#14150),
 .UNSPECIFIED.,.F.,.F.,(4,1,4),(0.283259011433087,4.63063308449434,10.4271318523291),
 .UNSPECIFIED.);
#264=B_SPLINE_CURVE_WITH_KNOTS('',3,(#14171,#14172,#14173,#14174),
 .UNSPECIFIED.,.F.,.F.,(4,4),(0.000779732613545348,0.618164468641375),
 .UNSPECIFIED.);
#265=B_SPLINE_CURVE_WITH_KNOTS('',3,(#14175,#14176,#14177,#14178),
 .UNSPECIFIED.,.F.,.F.,(4,4),(-0.618164468641375,-4.9439619065339E-17),
 .UNSPECIFIED.);
#266=B_SPLINE_CURVE_WITH_KNOTS('',3,(#14199,#14200,#14201,#14202),
 .UNSPECIFIED.,.F.,.F.,(4,4),(3.0964814046186E-16,0.618164468641375),
 .UNSPECIFIED.);
#267=B_SPLINE_CURVE_WITH_KNOTS('',3,(#14203,#14204,#14205,#14206),
 .UNSPECIFIED.,.F.,.F.,(4,4),(-0.618164468641375,-0.0007797326135453),
 .UNSPECIFIED.);
#268=B_SPLINE_CURVE_WITH_KNOTS('',3,(#14232,#14233,#14234,#14235,#14236),
 .UNSPECIFIED.,.F.,.F.,(4,1,4),(-10.419271481025,-4.62277271319024,-0.27539863731415),
 .UNSPECIFIED.);
#269=B_SPLINE_CURVE_WITH_KNOTS('',3,(#14237,#14238,#14239,#14240,#14241),
 .UNSPECIFIED.,.F.,.F.,(4,1,4),(0.27539863731415,4.62277271319024,10.419271481025),
 .UNSPECIFIED.);
#270=B_SPLINE_CURVE_WITH_KNOTS('',3,(#14262,#14263,#14264,#14265),
 .UNSPECIFIED.,.F.,.F.,(4,4),(0.00110654915602046,0.618489359031386),
 .UNSPECIFIED.);
#271=B_SPLINE_CURVE_WITH_KNOTS('',3,(#14266,#14267,#14268,#14269),
 .UNSPECIFIED.,.F.,.F.,(4,4),(-0.618489359031386,6.93889390390723E-18),
 .UNSPECIFIED.);
#557=SHAPE_REPRESENTATION_RELATIONSHIP('SRR','None',#22177,#566);
#566=ADVANCED_BREP_SHAPE_REPRESENTATION('',(#584),#22123);
#575=STYLED_ITEM('',(#22235),#584);
#584=MANIFOLD_SOLID_BREP('Body1',#8806);
#599=FACE_BOUND('',#1551,.T.);
#600=FACE_BOUND('',#1552,.T.);
#601=FACE_BOUND('',#1553,.T.);
#602=FACE_BOUND('',#1560,.T.);
#603=FACE_BOUND('',#1563,.T.);
#604=FACE_BOUND('',#1574,.T.);
#605=FACE_BOUND('',#1576,.T.);
#606=FACE_BOUND('',#1588,.T.);
#607=FACE_BOUND('',#1609,.T.);
#608=FACE_BOUND('',#1610,.T.);
#609=FACE_BOUND('',#1611,.T.);
#610=FACE_BOUND('',#1646,.T.);
#611=FACE_BOUND('',#1647,.T.);
#612=FACE_BOUND('',#1648,.T.);
#613=FACE_BOUND('',#1649,.T.);
#614=FACE_BOUND('',#1650,.T.);
#615=FACE_BOUND('',#1651,.T.);
#789=PLANE('',#9097);
#790=PLANE('',#9114);
#791=PLANE('',#9119);
#792=PLANE('',#9125);
#793=PLANE('',#9126);
#794=PLANE('',#9127);
#795=PLANE('',#9128);
#796=PLANE('',#9129);
#797=PLANE('',#9130);
#798=PLANE('',#9131);
#799=PLANE('',#9132);
#800=PLANE('',#9134);
#801=PLANE('',#9136);
#802=PLANE('',#9137);
#803=PLANE('',#9138);
#804=PLANE('',#9139);
#805=PLANE('',#9140);
#806=PLANE('',#9141);
#807=PLANE('',#9142);
#808=PLANE('',#9143);
#809=PLANE('',#9144);
#810=PLANE('',#9145);
#811=PLANE('',#9146);
#812=PLANE('',#9150);
#813=PLANE('',#9152);
#814=PLANE('',#9153);
#815=PLANE('',#9154);
#816=PLANE('',#9155);
#817=PLANE('',#9156);
#818=PLANE('',#9157);
#819=PLANE('',#9159);
#820=PLANE('',#9176);
#821=PLANE('',#9195);
#822=PLANE('',#9196);
#823=PLANE('',#9197);
#1052=FACE_OUTER_BOUND('',#1544,.T.);
#1053=FACE_OUTER_BOUND('',#1545,.T.);
#1054=FACE_OUTER_BOUND('',#1546,.T.);
#1055=FACE_OUTER_BOUND('',#1547,.T.);
#1056=FACE_OUTER_BOUND('',#1548,.T.);
#1057=FACE_OUTER_BOUND('',#1549,.T.);
#1058=FACE_OUTER_BOUND('',#1550,.T.);
#1059=FACE_OUTER_BOUND('',#1554,.T.);
#1060=FACE_OUTER_BOUND('',#1555,.T.);
#1061=FACE_OUTER_BOUND('',#1556,.T.);
#1062=FACE_OUTER_BOUND('',#1557,.T.);
#1063=FACE_OUTER_BOUND('',#1558,.T.);
#1064=FACE_OUTER_BOUND('',#1559,.T.);
#1065=FACE_OUTER_BOUND('',#1561,.T.);
#1066=FACE_OUTER_BOUND('',#1562,.T.);
#1067=FACE_OUTER_BOUND('',#1564,.T.);
#1068=FACE_OUTER_BOUND('',#1565,.T.);
#1069=FACE_OUTER_BOUND('',#1566,.T.);
#1070=FACE_OUTER_BOUND('',#1567,.T.);
#1071=FACE_OUTER_BOUND('',#1568,.T.);
#1072=FACE_OUTER_BOUND('',#1569,.T.);
#1073=FACE_OUTER_BOUND('',#1570,.T.);
#1074=FACE_OUTER_BOUND('',#1571,.T.);
#1075=FACE_OUTER_BOUND('',#1572,.T.);
#1076=FACE_OUTER_BOUND('',#1573,.T.);
#1077=FACE_OUTER_BOUND('',#1575,.T.);
#1078=FACE_OUTER_BOUND('',#1577,.T.);
#1079=FACE_OUTER_BOUND('',#1578,.T.);
#1080=FACE_OUTER_BOUND('',#1579,.T.);
#1081=FACE_OUTER_BOUND('',#1580,.T.);
#1082=FACE_OUTER_BOUND('',#1581,.T.);
#1083=FACE_OUTER_BOUND('',#1582,.T.);
#1084=FACE_OUTER_BOUND('',#1583,.T.);
#1085=FACE_OUTER_BOUND('',#1584,.T.);
#1086=FACE_OUTER_BOUND('',#1585,.T.);
#1087=FACE_OUTER_BOUND('',#1586,.T.);
#1088=FACE_OUTER_BOUND('',#1587,.T.);
#1089=FACE_OUTER_BOUND('',#1589,.T.);
#1090=FACE_OUTER_BOUND('',#1590,.T.);
#1091=FACE_OUTER_BOUND('',#1591,.T.);
#1092=FACE_OUTER_BOUND('',#1592,.T.);
#1093=FACE_OUTER_BOUND('',#1593,.T.);
#1094=FACE_OUTER_BOUND('',#1594,.T.);
#1095=FACE_OUTER_BOUND('',#1595,.T.);
#1096=FACE_OUTER_BOUND('',#1596,.T.);
#1097=FACE_OUTER_BOUND('',#1597,.T.);
#1098=FACE_OUTER_BOUND('',#1598,.T.);
#1099=FACE_OUTER_BOUND('',#1599,.T.);
#1100=FACE_OUTER_BOUND('',#1600,.T.);
#1101=FACE_OUTER_BOUND('',#1601,.T.);
#1102=FACE_OUTER_BOUND('',#1602,.T.);
#1103=FACE_OUTER_BOUND('',#1603,.T.);
#1104=FACE_OUTER_BOUND('',#1604,.T.);
#1105=FACE_OUTER_BOUND('',#1605,.T.);
#1106=FACE_OUTER_BOUND('',#1606,.T.);
#1107=FACE_OUTER_BOUND('',#1607,.T.);
#1108=FACE_OUTER_BOUND('',#1608,.T.);
#1109=FACE_OUTER_BOUND('',#1612,.T.);
#1110=FACE_OUTER_BOUND('',#1613,.T.);
#1111=FACE_OUTER_BOUND('',#1614,.T.);
#1112=FACE_OUTER_BOUND('',#1615,.T.);
#1113=FACE_OUTER_BOUND('',#1616,.T.);
#1114=FACE_OUTER_BOUND('',#1617,.T.);
#1115=FACE_OUTER_BOUND('',#1618,.T.);
#1116=FACE_OUTER_BOUND('',#1619,.T.);
#1117=FACE_OUTER_BOUND('',#1620,.T.);
#1118=FACE_OUTER_BOUND('',#1621,.T.);
#1119=FACE_OUTER_BOUND('',#1622,.T.);
#1120=FACE_OUTER_BOUND('',#1623,.T.);
#1121=FACE_OUTER_BOUND('',#1624,.T.);
#1122=FACE_OUTER_BOUND('',#1625,.T.);
#1123=FACE_OUTER_BOUND('',#1626,.T.);
#1124=FACE_OUTER_BOUND('',#1627,.T.);
#1125=FACE_OUTER_BOUND('',#1628,.T.);
#1126=FACE_OUTER_BOUND('',#1629,.T.);
#1127=FACE_OUTER_BOUND('',#1630,.T.);
#1128=FACE_OUTER_BOUND('',#1631,.T.);
#1129=FACE_OUTER_BOUND('',#1632,.T.);
#1130=FACE_OUTER_BOUND('',#1633,.T.);
#1131=FACE_OUTER_BOUND('',#1634,.T.);
#1132=FACE_OUTER_BOUND('',#1635,.T.);
#1133=FACE_OUTER_BOUND('',#1636,.T.);
#1134=FACE_OUTER_BOUND('',#1637,.T.);
#1135=FACE_OUTER_BOUND('',#1638,.T.);
#1136=FACE_OUTER_BOUND('',#1639,.T.);
#1137=FACE_OUTER_BOUND('',#1640,.T.);
#1138=FACE_OUTER_BOUND('',#1641,.T.);
#1139=FACE_OUTER_BOUND('',#1642,.T.);
#1140=FACE_OUTER_BOUND('',#1643,.T.);
#1141=FACE_OUTER_BOUND('',#1644,.T.);
#1142=FACE_OUTER_BOUND('',#1645,.T.);
#1143=FACE_OUTER_BOUND('',#1652,.T.);
#1144=FACE_OUTER_BOUND('',#1653,.T.);
#1544=EDGE_LOOP('',(#6486,#6487));
#1545=EDGE_LOOP('',(#6488,#6489));
#1546=EDGE_LOOP('',(#6490,#6491));
#1547=EDGE_LOOP('',(#6492,#6493));
#1548=EDGE_LOOP('',(#6494,#6495,#6496,#6497,#6498,#6499));
#1549=EDGE_LOOP('',(#6500,#6501,#6502,#6503,#6504,#6505));
#1550=EDGE_LOOP('',(#6506,#6507,#6508,#6509,#6510,#6511,#6512,#6513));
#1551=EDGE_LOOP('',(#6514));
#1552=EDGE_LOOP('',(#6515));
#1553=EDGE_LOOP('',(#6516));
#1554=EDGE_LOOP('',(#6517,#6518,#6519,#6520));
#1555=EDGE_LOOP('',(#6521,#6522,#6523,#6524));
#1556=EDGE_LOOP('',(#6525,#6526,#6527,#6528));
#1557=EDGE_LOOP('',(#6529,#6530,#6531,#6532));
#1558=EDGE_LOOP('',(#6533,#6534,#6535,#6536));
#1559=EDGE_LOOP('',(#6537));
#1560=EDGE_LOOP('',(#6538));
#1561=EDGE_LOOP('',(#6539,#6540,#6541,#6542));
#1562=EDGE_LOOP('',(#6543));
#1563=EDGE_LOOP('',(#6544));
#1564=EDGE_LOOP('',(#6545,#6546,#6547,#6548));
#1565=EDGE_LOOP('',(#6549,#6550,#6551,#6552));
#1566=EDGE_LOOP('',(#6553,#6554,#6555,#6556));
#1567=EDGE_LOOP('',(#6557,#6558,#6559,#6560));
#1568=EDGE_LOOP('',(#6561,#6562,#6563,#6564));
#1569=EDGE_LOOP('',(#6565,#6566,#6567,#6568));
#1570=EDGE_LOOP('',(#6569,#6570,#6571,#6572));
#1571=EDGE_LOOP('',(#6573,#6574,#6575,#6576));
#1572=EDGE_LOOP('',(#6577,#6578,#6579,#6580));
#1573=EDGE_LOOP('',(#6581));
#1574=EDGE_LOOP('',(#6582));
#1575=EDGE_LOOP('',(#6583));
#1576=EDGE_LOOP('',(#6584));
#1577=EDGE_LOOP('',(#6585,#6586,#6587,#6588));
#1578=EDGE_LOOP('',(#6589,#6590,#6591,#6592));
#1579=EDGE_LOOP('',(#6593,#6594,#6595,#6596));
#1580=EDGE_LOOP('',(#6597,#6598,#6599,#6600));
#1581=EDGE_LOOP('',(#6601,#6602,#6603,#6604));
#1582=EDGE_LOOP('',(#6605,#6606,#6607,#6608,#6609,#6610));
#1583=EDGE_LOOP('',(#6611,#6612,#6613,#6614,#6615,#6616,#6617,#6618,#6619,
#6620));
#1584=EDGE_LOOP('',(#6621,#6622,#6623,#6624,#6625,#6626,#6627,#6628,#6629,
#6630));
#1585=EDGE_LOOP('',(#6631,#6632,#6633,#6634,#6635,#6636,#6637,#6638,#6639,
#6640));
#1586=EDGE_LOOP('',(#6641,#6642,#6643,#6644,#6645,#6646,#6647,#6648));
#1587=EDGE_LOOP('',(#6649,#6650,#6651,#6652,#6653,#6654,#6655,#6656,#6657,
#6658,#6659,#6660,#6661,#6662,#6663,#6664,#6665,#6666,#6667,#6668,#6669,
#6670,#6671,#6672,#6673,#6674,#6675,#6676,#6677,#6678,#6679,#6680,#6681,
#6682,#6683,#6684,#6685,#6686,#6687,#6688,#6689,#6690));
#1588=EDGE_LOOP('',(#6691,#6692,#6693,#6694,#6695,#6696));
#1589=EDGE_LOOP('',(#6697,#6698,#6699,#6700));
#1590=EDGE_LOOP('',(#6701,#6702,#6703,#6704));
#1591=EDGE_LOOP('',(#6705,#6706,#6707,#6708,#6709,#6710));
#1592=EDGE_LOOP('',(#6711,#6712,#6713,#6714));
#1593=EDGE_LOOP('',(#6715,#6716,#6717,#6718));
#1594=EDGE_LOOP('',(#6719,#6720,#6721,#6722,#6723,#6724));
#1595=EDGE_LOOP('',(#6725,#6726,#6727,#6728));
#1596=EDGE_LOOP('',(#6729,#6730,#6731,#6732));
#1597=EDGE_LOOP('',(#6733,#6734,#6735,#6736));
#1598=EDGE_LOOP('',(#6737,#6738,#6739,#6740));
#1599=EDGE_LOOP('',(#6741,#6742,#6743,#6744,#6745,#6746,#6747,#6748,#6749,
#6750));
#1600=EDGE_LOOP('',(#6751,#6752,#6753,#6754));
#1601=EDGE_LOOP('',(#6755,#6756,#6757,#6758));
#1602=EDGE_LOOP('',(#6759,#6760,#6761,#6762));
#1603=EDGE_LOOP('',(#6763,#6764,#6765,#6766));
#1604=EDGE_LOOP('',(#6767,#6768,#6769,#6770));
#1605=EDGE_LOOP('',(#6771,#6772,#6773,#6774,#6775,#6776,#6777,#6778,#6779,
#6780));
#1606=EDGE_LOOP('',(#6781,#6782,#6783,#6784));
#1607=EDGE_LOOP('',(#6785,#6786,#6787,#6788,#6789,#6790));
#1608=EDGE_LOOP('',(#6791,#6792,#6793,#6794,#6795,#6796,#6797,#6798));
#1609=EDGE_LOOP('',(#6799));
#1610=EDGE_LOOP('',(#6800));
#1611=EDGE_LOOP('',(#6801));
#1612=EDGE_LOOP('',(#6802,#6803,#6804,#6805));
#1613=EDGE_LOOP('',(#6806,#6807,#6808,#6809,#6810,#6811,#6812,#6813,#6814,
#6815));
#1614=EDGE_LOOP('',(#6816,#6817,#6818,#6819));
#1615=EDGE_LOOP('',(#6820,#6821,#6822,#6823));
#1616=EDGE_LOOP('',(#6824,#6825,#6826,#6827));
#1617=EDGE_LOOP('',(#6828,#6829,#6830,#6831));
#1618=EDGE_LOOP('',(#6832,#6833,#6834,#6835));
#1619=EDGE_LOOP('',(#6836,#6837,#6838));
#1620=EDGE_LOOP('',(#6839,#6840,#6841));
#1621=EDGE_LOOP('',(#6842,#6843,#6844));
#1622=EDGE_LOOP('',(#6845,#6846,#6847,#6848));
#1623=EDGE_LOOP('',(#6849,#6850,#6851,#6852));
#1624=EDGE_LOOP('',(#6853,#6854,#6855));
#1625=EDGE_LOOP('',(#6856,#6857,#6858,#6859));
#1626=EDGE_LOOP('',(#6860,#6861,#6862,#6863));
#1627=EDGE_LOOP('',(#6864,#6865,#6866,#6867));
#1628=EDGE_LOOP('',(#6868,#6869,#6870,#6871));
#1629=EDGE_LOOP('',(#6872,#6873,#6874,#6875));
#1630=EDGE_LOOP('',(#6876,#6877,#6878,#6879));
#1631=EDGE_LOOP('',(#6880,#6881,#6882));
#1632=EDGE_LOOP('',(#6883,#6884,#6885));
#1633=EDGE_LOOP('',(#6886,#6887,#6888));
#1634=EDGE_LOOP('',(#6889,#6890,#6891,#6892));
#1635=EDGE_LOOP('',(#6893,#6894,#6895,#6896));
#1636=EDGE_LOOP('',(#6897,#6898,#6899));
#1637=EDGE_LOOP('',(#6900,#6901,#6902,#6903));
#1638=EDGE_LOOP('',(#6904,#6905,#6906,#6907));
#1639=EDGE_LOOP('',(#6908,#6909,#6910,#6911));
#1640=EDGE_LOOP('',(#6912,#6913,#6914,#6915));
#1641=EDGE_LOOP('',(#6916,#6917,#6918,#6919));
#1642=EDGE_LOOP('',(#6920,#6921,#6922,#6923));
#1643=EDGE_LOOP('',(#6924,#6925,#6926,#6927));
#1644=EDGE_LOOP('',(#6928,#6929,#6930,#6931,#6932,#6933,#6934,#6935));
#1645=EDGE_LOOP('',(#6936,#6937,#6938,#6939));
#1646=EDGE_LOOP('',(#6940));
#1647=EDGE_LOOP('',(#6941));
#1648=EDGE_LOOP('',(#6942));
#1649=EDGE_LOOP('',(#6943));
#1650=EDGE_LOOP('',(#6944));
#1651=EDGE_LOOP('',(#6945));
#1652=EDGE_LOOP('',(#6946,#6947,#6948,#6949));
#1653=EDGE_LOOP('',(#6950,#6951,#6952,#6953));
#2328=LINE('',#12555,#3058);
#2329=LINE('',#12557,#3059);
#2330=LINE('',#12571,#3060);
#2331=LINE('',#12576,#3061);
#2332=LINE('',#12582,#3062);
#2333=LINE('',#12587,#3063);
#2334=LINE('',#12592,#3064);
#2335=LINE('',#12601,#3065);
#2336=LINE('',#12608,#3066);
#2337=LINE('',#12612,#3067);
#2338=LINE('',#12617,#3068);
#2339=LINE('',#12619,#3069);
#2340=LINE('',#12621,#3070);
#2341=LINE('',#12622,#3071);
#2342=LINE('',#12626,#3072);
#2343=LINE('',#12628,#3073);
#2344=LINE('',#12630,#3074);
#2345=LINE('',#12631,#3075);
#2346=LINE('',#12635,#3076);
#2347=LINE('',#12637,#3077);
#2348=LINE('',#12639,#3078);
#2349=LINE('',#12640,#3079);
#2350=LINE('',#12644,#3080);
#2351=LINE('',#12646,#3081);
#2352=LINE('',#12648,#3082);
#2353=LINE('',#12649,#3083);
#2354=LINE('',#12653,#3084);
#2355=LINE('',#12655,#3085);
#2356=LINE('',#12657,#3086);
#2357=LINE('',#12658,#3087);
#2358=LINE('',#12662,#3088);
#2359=LINE('',#12664,#3089);
#2360=LINE('',#12666,#3090);
#2361=LINE('',#12667,#3091);
#2362=LINE('',#12671,#3092);
#2363=LINE('',#12673,#3093);
#2364=LINE('',#12675,#3094);
#2365=LINE('',#12676,#3095);
#2366=LINE('',#12684,#3096);
#2367=LINE('',#12685,#3097);
#2368=LINE('',#12687,#3098);
#2369=LINE('',#12688,#3099);
#2370=LINE('',#12690,#3100);
#2371=LINE('',#12691,#3101);
#2372=LINE('',#12694,#3102);
#2373=LINE('',#12696,#3103);
#2374=LINE('',#12697,#3104);
#2375=LINE('',#12700,#3105);
#2376=LINE('',#12702,#3106);
#2377=LINE('',#12703,#3107);
#2378=LINE('',#12707,#3108);
#2379=LINE('',#12751,#3109);
#2380=LINE('',#12794,#3110);
#2381=LINE('',#12797,#3111);
#2382=LINE('',#12835,#3112);
#2383=LINE('',#12872,#3113);
#2384=LINE('',#12875,#3114);
#2385=LINE('',#12883,#3115);
#2386=LINE('',#12920,#3116);
#2387=LINE('',#12923,#3117);
#2388=LINE('',#12930,#3118);
#2389=LINE('',#12936,#3119);
#2390=LINE('',#12947,#3120);
#2391=LINE('',#12956,#3121);
#2392=LINE('',#12962,#3122);
#2393=LINE('',#12997,#3123);
#2394=LINE('',#13068,#3124);
#2395=LINE('',#13138,#3125);
#2396=LINE('',#13170,#3126);
#2397=LINE('',#13176,#3127);
#2398=LINE('',#13185,#3128);
#2399=LINE('',#13222,#3129);
#2400=LINE('',#13257,#3130);
#2401=LINE('',#13259,#3131);
#2402=LINE('',#13263,#3132);
#2403=LINE('',#13309,#3133);
#2404=LINE('',#13435,#3134);
#2405=LINE('',#13515,#3135);
#2406=LINE('',#13677,#3136);
#2407=LINE('',#13787,#3137);
#2408=LINE('',#13876,#3138);
#2409=LINE('',#13964,#3139);
#2410=LINE('',#14076,#3140);
#2411=LINE('',#14077,#3141);
#2412=LINE('',#14114,#3142);
#2413=LINE('',#14115,#3143);
#3058=VECTOR('',#10270,1.);
#3059=VECTOR('',#10271,1.);
#3060=VECTOR('',#10282,0.15);
#3061=VECTOR('',#10287,0.15);
#3062=VECTOR('',#10294,0.15);
#3063=VECTOR('',#10301,0.15);
#3064=VECTOR('',#10306,0.3);
#3065=VECTOR('',#10317,0.3);
#3066=VECTOR('',#10326,0.17);
#3067=VECTOR('',#10331,0.17);
#3068=VECTOR('',#10336,1.);
#3069=VECTOR('',#10337,1.);
#3070=VECTOR('',#10338,1.);
#3071=VECTOR('',#10339,1.);
#3072=VECTOR('',#10342,1.);
#3073=VECTOR('',#10343,1.);
#3074=VECTOR('',#10344,1.);
#3075=VECTOR('',#10345,1.);
#3076=VECTOR('',#10348,1.);
#3077=VECTOR('',#10349,1.);
#3078=VECTOR('',#10350,1.);
#3079=VECTOR('',#10351,1.);
#3080=VECTOR('',#10354,1.);
#3081=VECTOR('',#10355,1.);
#3082=VECTOR('',#10356,1.);
#3083=VECTOR('',#10357,1.);
#3084=VECTOR('',#10360,1.);
#3085=VECTOR('',#10361,1.);
#3086=VECTOR('',#10362,1.);
#3087=VECTOR('',#10363,1.);
#3088=VECTOR('',#10366,1.);
#3089=VECTOR('',#10367,1.);
#3090=VECTOR('',#10368,1.);
#3091=VECTOR('',#10369,1.);
#3092=VECTOR('',#10372,1.);
#3093=VECTOR('',#10373,1.);
#3094=VECTOR('',#10374,1.);
#3095=VECTOR('',#10375,1.);
#3096=VECTOR('',#10386,1.);
#3097=VECTOR('',#10387,1.);
#3098=VECTOR('',#10390,1.);
#3099=VECTOR('',#10391,1.);
#3100=VECTOR('',#10394,1.);
#3101=VECTOR('',#10395,1.);
#3102=VECTOR('',#10398,1.);
#3103=VECTOR('',#10399,1.);
#3104=VECTOR('',#10400,1.);
#3105=VECTOR('',#10403,1.);
#3106=VECTOR('',#10404,1.);
#3107=VECTOR('',#10405,1.);
#3108=VECTOR('',#10408,1.);
#3109=VECTOR('',#10411,1.);
#3110=VECTOR('',#10412,1.);
#3111=VECTOR('',#10415,1.);
#3112=VECTOR('',#10416,1.);
#3113=VECTOR('',#10417,1.);
#3114=VECTOR('',#10420,1.);
#3115=VECTOR('',#10421,1.);
#3116=VECTOR('',#10422,1.);
#3117=VECTOR('',#10425,1.);
#3118=VECTOR('',#10426,1.);
#3119=VECTOR('',#10427,1.);
#3120=VECTOR('',#10430,1.);
#3121=VECTOR('',#10431,1.);
#3122=VECTOR('',#10432,1.);
#3123=VECTOR('',#10433,1.);
#3124=VECTOR('',#10434,1.);
#3125=VECTOR('',#10435,1.);
#3126=VECTOR('',#10436,1.);
#3127=VECTOR('',#10437,1.);
#3128=VECTOR('',#10438,1.);
#3129=VECTOR('',#10439,1.);
#3130=VECTOR('',#10440,1.);
#3131=VECTOR('',#10443,0.4);
#3132=VECTOR('',#10448,0.4);
#3133=VECTOR('',#10451,1.);
#3134=VECTOR('',#10456,1.);
#3135=VECTOR('',#10459,1.);
#3136=VECTOR('',#10464,1.);
#3137=VECTOR('',#10469,1.);
#3138=VECTOR('',#10474,1.);
#3139=VECTOR('',#10507,1.);
#3140=VECTOR('',#10536,1.);
#3141=VECTOR('',#10537,1.);
#3142=VECTOR('',#10548,1.);
#3143=VECTOR('',#10549,1.);
#3412=CIRCLE('',#9090,0.25);
#3413=CIRCLE('',#9092,0.25);
#3414=CIRCLE('',#9094,0.25);
#3415=CIRCLE('',#9096,0.25);
#3416=CIRCLE('',#9098,0.15);
#3417=CIRCLE('',#9099,0.15);
#3418=CIRCLE('',#9100,0.4);
#3419=CIRCLE('',#9102,0.15);
#3420=CIRCLE('',#9104,0.15);
#3421=CIRCLE('',#9105,0.15);
#3422=CIRCLE('',#9107,0.15);
#3423=CIRCLE('',#9108,0.15);
#3424=CIRCLE('',#9110,0.15);
#3425=CIRCLE('',#9112,0.3);
#3426=CIRCLE('',#9113,0.3);
#3427=CIRCLE('',#9115,0.17);
#3428=CIRCLE('',#9117,0.3);
#3429=CIRCLE('',#9118,0.3);
#3430=CIRCLE('',#9120,0.17);
#3431=CIRCLE('',#9122,0.17);
#3432=CIRCLE('',#9124,0.17);
#3433=CIRCLE('',#9133,0.4);
#3434=CIRCLE('',#9135,0.4);
#3435=CIRCLE('',#9149,0.4);
#3436=CIRCLE('',#9151,0.1);
#3437=CIRCLE('',#9158,0.0999999999999995);
#3438=CIRCLE('',#9160,0.1);
#3439=CIRCLE('',#9162,0.1);
#3440=CIRCLE('',#9163,0.1);
#3441=CIRCLE('',#9165,0.0999999999999999);
#3442=CIRCLE('',#9166,0.0999999999999998);
#3443=CIRCLE('',#9167,0.0999999999999998);
#3444=CIRCLE('',#9169,0.0999999999999994);
#3445=CIRCLE('',#9170,0.0999999999999993);
#3446=CIRCLE('',#9173,0.0999999999999999);
#3447=CIRCLE('',#9174,0.1);
#3448=CIRCLE('',#9178,0.3);
#3449=CIRCLE('',#9179,0.3);
#3450=CIRCLE('',#9180,0.3);
#3451=CIRCLE('',#9182,0.3);
#3452=CIRCLE('',#9183,0.3);
#3453=CIRCLE('',#9184,0.3);
#3454=CIRCLE('',#9186,0.3);
#3455=CIRCLE('',#9187,0.299999999999999);
#3456=CIRCLE('',#9188,0.3);
#3457=CIRCLE('',#9191,0.3);
#3458=CIRCLE('',#9192,0.3);
#3459=CIRCLE('',#9193,0.3);
#3828=VERTEX_POINT('',#12262);
#3829=VERTEX_POINT('',#12263);
#3830=VERTEX_POINT('',#12290);
#3831=VERTEX_POINT('',#12291);
#3832=VERTEX_POINT('',#12314);
#3833=VERTEX_POINT('',#12315);
#3834=VERTEX_POINT('',#12338);
#3835=VERTEX_POINT('',#12339);
#3836=VERTEX_POINT('',#12385);
#3837=VERTEX_POINT('',#12390);
#3838=VERTEX_POINT('',#12419);
#3839=VERTEX_POINT('',#12424);
#3840=VERTEX_POINT('',#12477);
#3841=VERTEX_POINT('',#12482);
#3842=VERTEX_POINT('',#12511);
#3843=VERTEX_POINT('',#12516);
#3844=VERTEX_POINT('',#12550);
#3845=VERTEX_POINT('',#12556);
#3846=VERTEX_POINT('',#12562);
#3847=VERTEX_POINT('',#12564);
#3848=VERTEX_POINT('',#12566);
#3849=VERTEX_POINT('',#12569);
#3850=VERTEX_POINT('',#12573);
#3851=VERTEX_POINT('',#12575);
#3852=VERTEX_POINT('',#12579);
#3853=VERTEX_POINT('',#12581);
#3854=VERTEX_POINT('',#12585);
#3855=VERTEX_POINT('',#12589);
#3856=VERTEX_POINT('',#12591);
#3857=VERTEX_POINT('',#12595);
#3858=VERTEX_POINT('',#12598);
#3859=VERTEX_POINT('',#12600);
#3860=VERTEX_POINT('',#12604);
#3861=VERTEX_POINT('',#12607);
#3862=VERTEX_POINT('',#12611);
#3863=VERTEX_POINT('',#12615);
#3864=VERTEX_POINT('',#12616);
#3865=VERTEX_POINT('',#12618);
#3866=VERTEX_POINT('',#12620);
#3867=VERTEX_POINT('',#12624);
#3868=VERTEX_POINT('',#12625);
#3869=VERTEX_POINT('',#12627);
#3870=VERTEX_POINT('',#12629);
#3871=VERTEX_POINT('',#12633);
#3872=VERTEX_POINT('',#12634);
#3873=VERTEX_POINT('',#12636);
#3874=VERTEX_POINT('',#12638);
#3875=VERTEX_POINT('',#12642);
#3876=VERTEX_POINT('',#12643);
#3877=VERTEX_POINT('',#12645);
#3878=VERTEX_POINT('',#12647);
#3879=VERTEX_POINT('',#12651);
#3880=VERTEX_POINT('',#12652);
#3881=VERTEX_POINT('',#12654);
#3882=VERTEX_POINT('',#12656);
#3883=VERTEX_POINT('',#12660);
#3884=VERTEX_POINT('',#12661);
#3885=VERTEX_POINT('',#12663);
#3886=VERTEX_POINT('',#12665);
#3887=VERTEX_POINT('',#12669);
#3888=VERTEX_POINT('',#12670);
#3889=VERTEX_POINT('',#12672);
#3890=VERTEX_POINT('',#12674);
#3891=VERTEX_POINT('',#12678);
#3892=VERTEX_POINT('',#12681);
#3893=VERTEX_POINT('',#12693);
#3894=VERTEX_POINT('',#12695);
#3895=VERTEX_POINT('',#12699);
#3896=VERTEX_POINT('',#12701);
#3897=VERTEX_POINT('',#12705);
#3898=VERTEX_POINT('',#12706);
#3899=VERTEX_POINT('',#12708);
#3900=VERTEX_POINT('',#12750);
#3901=VERTEX_POINT('',#12758);
#3902=VERTEX_POINT('',#12787);
#3903=VERTEX_POINT('',#12796);
#3904=VERTEX_POINT('',#12798);
#3905=VERTEX_POINT('',#12805);
#3906=VERTEX_POINT('',#12834);
#3907=VERTEX_POINT('',#12836);
#3908=VERTEX_POINT('',#12865);
#3909=VERTEX_POINT('',#12874);
#3910=VERTEX_POINT('',#12882);
#3911=VERTEX_POINT('',#12884);
#3912=VERTEX_POINT('',#12913);
#3913=VERTEX_POINT('',#12922);
#3914=VERTEX_POINT('',#12924);
#3915=VERTEX_POINT('',#12929);
#3916=VERTEX_POINT('',#12931);
#3917=VERTEX_POINT('',#12946);
#3918=VERTEX_POINT('',#12955);
#3919=VERTEX_POINT('',#12961);
#3920=VERTEX_POINT('',#12963);
#3921=VERTEX_POINT('',#12996);
#3922=VERTEX_POINT('',#12998);
#3923=VERTEX_POINT('',#13030);
#3924=VERTEX_POINT('',#13035);
#3925=VERTEX_POINT('',#13067);
#3926=VERTEX_POINT('',#13069);
#3927=VERTEX_POINT('',#13101);
#3928=VERTEX_POINT('',#13106);
#3929=VERTEX_POINT('',#13139);
#3930=VERTEX_POINT('',#13165);
#3931=VERTEX_POINT('',#13171);
#3932=VERTEX_POINT('',#13177);
#3933=VERTEX_POINT('',#13186);
#3934=VERTEX_POINT('',#13187);
#3935=VERTEX_POINT('',#13192);
#3936=VERTEX_POINT('',#13221);
#3937=VERTEX_POINT('',#13223);
#3938=VERTEX_POINT('',#13252);
#3939=VERTEX_POINT('',#13261);
#3940=VERTEX_POINT('',#13265);
#3941=VERTEX_POINT('',#13272);
#3942=VERTEX_POINT('',#13279);
#3943=VERTEX_POINT('',#13308);
#3944=VERTEX_POINT('',#13374);
#3945=VERTEX_POINT('',#13423);
#3946=VERTEX_POINT('',#13430);
#3947=VERTEX_POINT('',#13468);
#3948=VERTEX_POINT('',#13478);
#3949=VERTEX_POINT('',#13485);
#3950=VERTEX_POINT('',#13514);
#3951=VERTEX_POINT('',#13516);
#3952=VERTEX_POINT('',#13641);
#3953=VERTEX_POINT('',#13648);
#3954=VERTEX_POINT('',#13750);
#3955=VERTEX_POINT('',#13757);
#3956=VERTEX_POINT('',#13786);
#3957=VERTEX_POINT('',#13788);
#3958=VERTEX_POINT('',#13839);
#3959=VERTEX_POINT('',#13868);
#3960=VERTEX_POINT('',#13875);
#3961=VERTEX_POINT('',#13897);
#3962=VERTEX_POINT('',#13932);
#3963=VERTEX_POINT('',#13960);
#3964=VERTEX_POINT('',#14055);
#3965=VERTEX_POINT('',#14056);
#3966=VERTEX_POINT('',#14058);
#3967=VERTEX_POINT('',#14062);
#3968=VERTEX_POINT('',#14063);
#3969=VERTEX_POINT('',#14065);
#3970=VERTEX_POINT('',#14069);
#3971=VERTEX_POINT('',#14070);
#3972=VERTEX_POINT('',#14072);
#3973=VERTEX_POINT('',#14107);
#3974=VERTEX_POINT('',#14108);
#3975=VERTEX_POINT('',#14110);
#4796=EDGE_CURVE('',#3828,#3829,#172,.T.);
#4797=EDGE_CURVE('',#3828,#3829,#3412,.T.);
#4798=EDGE_CURVE('',#3830,#3831,#173,.T.);
#4799=EDGE_CURVE('',#3830,#3831,#3413,.T.);
#4800=EDGE_CURVE('',#3832,#3833,#174,.T.);
#4801=EDGE_CURVE('',#3832,#3833,#3414,.T.);
#4802=EDGE_CURVE('',#3834,#3835,#175,.T.);
#4803=EDGE_CURVE('',#3834,#3835,#3415,.T.);
#4804=EDGE_CURVE('',#3836,#3831,#176,.T.);
#4805=EDGE_CURVE('',#3836,#3837,#177,.T.);
#4806=EDGE_CURVE('',#3838,#3837,#178,.T.);
#4807=EDGE_CURVE('',#3838,#3839,#179,.T.);
#4808=EDGE_CURVE('',#3830,#3839,#180,.T.);
#4809=EDGE_CURVE('',#3840,#3835,#181,.T.);
#4810=EDGE_CURVE('',#3840,#3841,#182,.T.);
#4811=EDGE_CURVE('',#3842,#3841,#183,.T.);
#4812=EDGE_CURVE('',#3842,#3843,#184,.T.);
#4813=EDGE_CURVE('',#3834,#3843,#185,.T.);
#4814=EDGE_CURVE('',#3828,#3844,#186,.T.);
#4815=EDGE_CURVE('',#3844,#3840,#2328,.T.);
#4816=EDGE_CURVE('',#3843,#3845,#2329,.T.);
#4817=EDGE_CURVE('',#3845,#3829,#187,.T.);
#4818=EDGE_CURVE('',#3846,#3846,#3416,.T.);
#4819=EDGE_CURVE('',#3847,#3847,#3417,.T.);
#4820=EDGE_CURVE('',#3848,#3848,#3418,.T.);
#4821=EDGE_CURVE('',#3849,#3849,#3419,.T.);
#4822=EDGE_CURVE('',#3849,#3846,#2330,.T.);
#4823=EDGE_CURVE('',#3850,#3850,#3420,.T.);
#4824=EDGE_CURVE('',#3850,#3851,#2331,.T.);
#4825=EDGE_CURVE('',#3851,#3851,#3421,.T.);
#4826=EDGE_CURVE('',#3852,#3852,#3422,.T.);
#4827=EDGE_CURVE('',#3852,#3853,#2332,.T.);
#4828=EDGE_CURVE('',#3853,#3853,#3423,.T.);
#4829=EDGE_CURVE('',#3854,#3854,#3424,.T.);
#4830=EDGE_CURVE('',#3854,#3847,#2333,.T.);
#4831=EDGE_CURVE('',#3855,#3855,#3425,.T.);
#4832=EDGE_CURVE('',#3855,#3856,#2334,.T.);
#4833=EDGE_CURVE('',#3856,#3856,#3426,.T.);
#4834=EDGE_CURVE('',#3857,#3857,#3427,.T.);
#4835=EDGE_CURVE('',#3858,#3858,#3428,.T.);
#4836=EDGE_CURVE('',#3858,#3859,#2335,.T.);
#4837=EDGE_CURVE('',#3859,#3859,#3429,.T.);
#4838=EDGE_CURVE('',#3860,#3860,#3430,.T.);
#4839=EDGE_CURVE('',#3857,#3861,#2336,.T.);
#4840=EDGE_CURVE('',#3861,#3861,#3431,.T.);
#4841=EDGE_CURVE('',#3860,#3862,#2337,.T.);
#4842=EDGE_CURVE('',#3862,#3862,#3432,.T.);
#4843=EDGE_CURVE('',#3863,#3864,#2338,.T.);
#4844=EDGE_CURVE('',#3865,#3863,#2339,.T.);
#4845=EDGE_CURVE('',#3866,#3865,#2340,.T.);
#4846=EDGE_CURVE('',#3866,#3864,#2341,.T.);
#4847=EDGE_CURVE('',#3867,#3868,#2342,.T.);
#4848=EDGE_CURVE('',#3867,#3869,#2343,.T.);
#4849=EDGE_CURVE('',#3870,#3869,#2344,.T.);
#4850=EDGE_CURVE('',#3868,#3870,#2345,.T.);
#4851=EDGE_CURVE('',#3871,#3872,#2346,.T.);
#4852=EDGE_CURVE('',#3871,#3873,#2347,.T.);
#4853=EDGE_CURVE('',#3874,#3873,#2348,.T.);
#4854=EDGE_CURVE('',#3872,#3874,#2349,.T.);
#4855=EDGE_CURVE('',#3875,#3876,#2350,.T.);
#4856=EDGE_CURVE('',#3875,#3877,#2351,.T.);
#4857=EDGE_CURVE('',#3878,#3877,#2352,.T.);
#4858=EDGE_CURVE('',#3876,#3878,#2353,.T.);
#4859=EDGE_CURVE('',#3879,#3880,#2354,.T.);
#4860=EDGE_CURVE('',#3879,#3881,#2355,.T.);
#4861=EDGE_CURVE('',#3882,#3881,#2356,.T.);
#4862=EDGE_CURVE('',#3880,#3882,#2357,.T.);
#4863=EDGE_CURVE('',#3883,#3884,#2358,.T.);
#4864=EDGE_CURVE('',#3885,#3883,#2359,.T.);
#4865=EDGE_CURVE('',#3886,#3885,#2360,.T.);
#4866=EDGE_CURVE('',#3886,#3884,#2361,.T.);
#4867=EDGE_CURVE('',#3887,#3888,#2362,.T.);
#4868=EDGE_CURVE('',#3889,#3887,#2363,.T.);
#4869=EDGE_CURVE('',#3890,#3889,#2364,.T.);
#4870=EDGE_CURVE('',#3890,#3888,#2365,.T.);
#4871=EDGE_CURVE('',#3891,#3891,#3433,.T.);
#4872=EDGE_CURVE('',#3892,#3892,#3434,.T.);
#4873=EDGE_CURVE('',#3864,#3879,#2366,.T.);
#4874=EDGE_CURVE('',#3881,#3866,#2367,.T.);
#4875=EDGE_CURVE('',#3884,#3867,#2368,.T.);
#4876=EDGE_CURVE('',#3869,#3886,#2369,.T.);
#4877=EDGE_CURVE('',#3888,#3871,#2370,.T.);
#4878=EDGE_CURVE('',#3873,#3890,#2371,.T.);
#4879=EDGE_CURVE('',#3893,#3875,#2372,.T.);
#4880=EDGE_CURVE('',#3894,#3893,#2373,.T.);
#4881=EDGE_CURVE('',#3877,#3894,#2374,.T.);
#4882=EDGE_CURVE('',#3895,#3893,#2375,.T.);
#4883=EDGE_CURVE('',#3896,#3895,#2376,.T.);
#4884=EDGE_CURVE('',#3894,#3896,#2377,.T.);
#4885=EDGE_CURVE('',#3897,#3898,#2378,.T.);
#4886=EDGE_CURVE('',#3899,#3898,#188,.T.);
#4887=EDGE_CURVE('',#3845,#3899,#189,.T.);
#4888=EDGE_CURVE('',#3897,#3842,#190,.T.);
#4889=EDGE_CURVE('',#3896,#3900,#2379,.T.);
#4890=EDGE_CURVE('',#3841,#3900,#191,.T.);
#4891=EDGE_CURVE('',#3901,#3844,#192,.T.);
#4892=EDGE_CURVE('',#3902,#3901,#193,.T.);
#4893=EDGE_CURVE('',#3902,#3878,#2380,.T.);
#4894=EDGE_CURVE('',#3889,#3903,#2381,.T.);
#4895=EDGE_CURVE('',#3904,#3903,#194,.T.);
#4896=EDGE_CURVE('',#3905,#3904,#195,.T.);
#4897=EDGE_CURVE('',#3906,#3905,#2382,.T.);
#4898=EDGE_CURVE('',#3907,#3906,#196,.T.);
#4899=EDGE_CURVE('',#3908,#3907,#197,.T.);
#4900=EDGE_CURVE('',#3908,#3874,#2383,.T.);
#4901=EDGE_CURVE('',#3885,#3909,#2384,.T.);
#4902=EDGE_CURVE('',#3837,#3909,#198,.T.);
#4903=EDGE_CURVE('',#3910,#3836,#2385,.T.);
#4904=EDGE_CURVE('',#3911,#3910,#199,.T.);
#4905=EDGE_CURVE('',#3912,#3911,#200,.T.);
#4906=EDGE_CURVE('',#3912,#3870,#2386,.T.);
#4907=EDGE_CURVE('',#3913,#3880,#2387,.T.);
#4908=EDGE_CURVE('',#3913,#3914,#201,.T.);
#4909=EDGE_CURVE('',#3914,#3915,#2388,.T.);
#4910=EDGE_CURVE('',#3915,#3916,#202,.T.);
#4911=EDGE_CURVE('',#3863,#3916,#2389,.T.);
#4912=EDGE_CURVE('',#3902,#3898,#203,.T.);
#4913=EDGE_CURVE('',#3897,#3900,#204,.T.);
#4914=EDGE_CURVE('',#3917,#3895,#2390,.T.);
#4915=EDGE_CURVE('',#3917,#3903,#205,.T.);
#4916=EDGE_CURVE('',#3918,#3887,#2391,.T.);
#4917=EDGE_CURVE('',#3918,#3909,#206,.T.);
#4918=EDGE_CURVE('',#3919,#3883,#2392,.T.);
#4919=EDGE_CURVE('',#3919,#3920,#207,.T.);
#4920=EDGE_CURVE('',#3920,#3913,#208,.T.);
#4921=EDGE_CURVE('',#3882,#3921,#2393,.T.);
#4922=EDGE_CURVE('',#3922,#3921,#209,.T.);
#4923=EDGE_CURVE('',#3922,#3923,#210,.T.);
#4924=EDGE_CURVE('',#3924,#3923,#211,.T.);
#4925=EDGE_CURVE('',#3924,#3925,#2394,.T.);
#4926=EDGE_CURVE('',#3926,#3925,#212,.T.);
#4927=EDGE_CURVE('',#3926,#3927,#213,.T.);
#4928=EDGE_CURVE('',#3928,#3927,#214,.T.);
#4929=EDGE_CURVE('',#3928,#3865,#2395,.T.);
#4930=EDGE_CURVE('',#3916,#3929,#215,.T.);
#4931=EDGE_CURVE('',#3929,#3930,#216,.T.);
#4932=EDGE_CURVE('',#3868,#3930,#2396,.T.);
#4933=EDGE_CURVE('',#3912,#3931,#217,.T.);
#4934=EDGE_CURVE('',#3872,#3931,#2397,.T.);
#4935=EDGE_CURVE('',#3908,#3932,#218,.T.);
#4936=EDGE_CURVE('',#3876,#3932,#2398,.T.);
#4937=EDGE_CURVE('',#3933,#3934,#219,.T.);
#4938=EDGE_CURVE('',#3934,#3935,#220,.T.);
#4939=EDGE_CURVE('',#3935,#3936,#2399,.T.);
#4940=EDGE_CURVE('',#3936,#3937,#221,.T.);
#4941=EDGE_CURVE('',#3937,#3938,#222,.T.);
#4942=EDGE_CURVE('',#3933,#3938,#2400,.T.);
#4943=EDGE_CURVE('',#3848,#3892,#2401,.T.);
#4944=EDGE_CURVE('',#3939,#3939,#3435,.T.);
#4945=EDGE_CURVE('',#3939,#3891,#2402,.T.);
#4946=EDGE_CURVE('',#3933,#3940,#223,.T.);
#4947=EDGE_CURVE('',#3941,#3938,#224,.T.);
#4948=EDGE_CURVE('',#3942,#3941,#225,.T.);
#4949=EDGE_CURVE('',#3943,#3942,#2403,.T.);
#4950=EDGE_CURVE('',#3940,#3943,#226,.T.);
#4951=EDGE_CURVE('',#3901,#3899,#227,.T.);
#4952=EDGE_CURVE('',#3940,#3944,#228,.T.);
#4953=EDGE_CURVE('',#3944,#3934,#229,.T.);
#4954=EDGE_CURVE('',#3945,#3943,#230,.T.);
#4955=EDGE_CURVE('',#3944,#3945,#3436,.F.);
#4956=EDGE_CURVE('',#3942,#3946,#231,.T.);
#4957=EDGE_CURVE('',#3946,#3945,#2404,.T.);
#4958=EDGE_CURVE('',#3937,#3947,#232,.T.);
#4959=EDGE_CURVE('',#3947,#3941,#233,.T.);
#4960=EDGE_CURVE('',#3948,#3932,#234,.T.);
#4961=EDGE_CURVE('',#3949,#3948,#235,.T.);
#4962=EDGE_CURVE('',#3950,#3949,#2405,.T.);
#4963=EDGE_CURVE('',#3951,#3950,#236,.T.);
#4964=EDGE_CURVE('',#3917,#3951,#237,.T.);
#4965=EDGE_CURVE('',#3907,#3948,#238,.T.);
#4966=EDGE_CURVE('',#3949,#3906,#239,.T.);
#4967=EDGE_CURVE('',#3905,#3950,#240,.T.);
#4968=EDGE_CURVE('',#3951,#3904,#241,.T.);
#4969=EDGE_CURVE('',#3952,#3931,#242,.T.);
#4970=EDGE_CURVE('',#3953,#3952,#243,.T.);
#4971=EDGE_CURVE('',#3839,#3953,#2406,.T.);
#4972=EDGE_CURVE('',#3918,#3838,#244,.T.);
#4973=EDGE_CURVE('',#3911,#3952,#245,.T.);
#4974=EDGE_CURVE('',#3953,#3833,#246,.T.);
#4975=EDGE_CURVE('',#3832,#3910,#247,.T.);
#4976=EDGE_CURVE('',#3954,#3930,#248,.T.);
#4977=EDGE_CURVE('',#3955,#3954,#249,.T.);
#4978=EDGE_CURVE('',#3956,#3955,#2407,.T.);
#4979=EDGE_CURVE('',#3957,#3956,#250,.T.);
#4980=EDGE_CURVE('',#3919,#3957,#251,.T.);
#4981=EDGE_CURVE('',#3929,#3958,#252,.T.);
#4982=EDGE_CURVE('',#3958,#3954,#253,.T.);
#4983=EDGE_CURVE('',#3959,#3958,#3437,.F.);
#4984=EDGE_CURVE('',#3955,#3959,#254,.T.);
#4985=EDGE_CURVE('',#3959,#3960,#2408,.T.);
#4986=EDGE_CURVE('',#3960,#3956,#255,.T.);
#4987=EDGE_CURVE('',#3957,#3961,#256,.T.);
#4988=EDGE_CURVE('',#3961,#3920,#257,.T.);
#4989=EDGE_CURVE('',#3961,#3960,#3438,.F.);
#4990=EDGE_CURVE('',#3960,#3914,#3439,.F.);
#4991=EDGE_CURVE('',#3914,#3961,#3440,.F.);
#4992=EDGE_CURVE('',#3946,#3947,#3441,.F.);
#4993=EDGE_CURVE('',#3947,#3962,#3442,.F.);
#4994=EDGE_CURVE('',#3962,#3946,#3443,.F.);
#4995=EDGE_CURVE('',#3958,#3915,#3444,.F.);
#4996=EDGE_CURVE('',#3915,#3959,#3445,.F.);
#4997=EDGE_CURVE('',#3963,#3944,#3446,.F.);
#4998=EDGE_CURVE('',#3945,#3963,#3447,.F.);
#4999=EDGE_CURVE('',#3963,#3962,#2409,.T.);
#5000=EDGE_CURVE('',#3935,#3963,#258,.T.);
#5001=EDGE_CURVE('',#3962,#3936,#259,.T.);
#5002=EDGE_CURVE('',#3964,#3965,#3448,.F.);
#5003=EDGE_CURVE('',#3966,#3964,#3449,.F.);
#5004=EDGE_CURVE('',#3965,#3966,#3450,.F.);
#5005=EDGE_CURVE('',#3967,#3968,#3451,.F.);
#5006=EDGE_CURVE('',#3969,#3967,#3452,.F.);
#5007=EDGE_CURVE('',#3968,#3969,#3453,.F.);
#5008=EDGE_CURVE('',#3970,#3971,#3454,.F.);
#5009=EDGE_CURVE('',#3972,#3970,#3455,.F.);
#5010=EDGE_CURVE('',#3971,#3972,#3456,.F.);
#5011=EDGE_CURVE('',#3965,#3972,#2410,.T.);
#5012=EDGE_CURVE('',#3970,#3964,#2411,.T.);
#5013=EDGE_CURVE('',#3927,#3971,#260,.T.);
#5014=EDGE_CURVE('',#3972,#3928,#261,.T.);
#5015=EDGE_CURVE('',#3973,#3974,#3457,.F.);
#5016=EDGE_CURVE('',#3975,#3973,#3458,.F.);
#5017=EDGE_CURVE('',#3974,#3975,#3459,.F.);
#5018=EDGE_CURVE('',#3973,#3969,#2412,.T.);
#5019=EDGE_CURVE('',#3967,#3975,#2413,.T.);
#5020=EDGE_CURVE('',#3971,#3974,#262,.T.);
#5021=EDGE_CURVE('',#3975,#3970,#263,.T.);
#5022=EDGE_CURVE('',#3925,#3973,#264,.T.);
#5023=EDGE_CURVE('',#3974,#3926,#265,.T.);
#5024=EDGE_CURVE('',#3923,#3968,#266,.T.);
#5025=EDGE_CURVE('',#3969,#3924,#267,.T.);
#5026=EDGE_CURVE('',#3968,#3966,#268,.T.);
#5027=EDGE_CURVE('',#3964,#3967,#269,.T.);
#5028=EDGE_CURVE('',#3921,#3965,#270,.T.);
#5029=EDGE_CURVE('',#3966,#3922,#271,.T.);
#6486=ORIENTED_EDGE('',*,*,#4796,.F.);
#6487=ORIENTED_EDGE('',*,*,#4797,.T.);
#6488=ORIENTED_EDGE('',*,*,#4798,.F.);
#6489=ORIENTED_EDGE('',*,*,#4799,.T.);
#6490=ORIENTED_EDGE('',*,*,#4800,.F.);
#6491=ORIENTED_EDGE('',*,*,#4801,.T.);
#6492=ORIENTED_EDGE('',*,*,#4802,.F.);
#6493=ORIENTED_EDGE('',*,*,#4803,.T.);
#6494=ORIENTED_EDGE('',*,*,#4798,.T.);
#6495=ORIENTED_EDGE('',*,*,#4804,.F.);
#6496=ORIENTED_EDGE('',*,*,#4805,.T.);
#6497=ORIENTED_EDGE('',*,*,#4806,.F.);
#6498=ORIENTED_EDGE('',*,*,#4807,.T.);
#6499=ORIENTED_EDGE('',*,*,#4808,.F.);
#6500=ORIENTED_EDGE('',*,*,#4802,.T.);
#6501=ORIENTED_EDGE('',*,*,#4809,.F.);
#6502=ORIENTED_EDGE('',*,*,#4810,.T.);
#6503=ORIENTED_EDGE('',*,*,#4811,.F.);
#6504=ORIENTED_EDGE('',*,*,#4812,.T.);
#6505=ORIENTED_EDGE('',*,*,#4813,.F.);
#6506=ORIENTED_EDGE('',*,*,#4814,.T.);
#6507=ORIENTED_EDGE('',*,*,#4815,.T.);
#6508=ORIENTED_EDGE('',*,*,#4809,.T.);
#6509=ORIENTED_EDGE('',*,*,#4803,.F.);
#6510=ORIENTED_EDGE('',*,*,#4813,.T.);
#6511=ORIENTED_EDGE('',*,*,#4816,.T.);
#6512=ORIENTED_EDGE('',*,*,#4817,.T.);
#6513=ORIENTED_EDGE('',*,*,#4797,.F.);
#6514=ORIENTED_EDGE('',*,*,#4818,.T.);
#6515=ORIENTED_EDGE('',*,*,#4819,.T.);
#6516=ORIENTED_EDGE('',*,*,#4820,.T.);
#6517=ORIENTED_EDGE('',*,*,#4821,.F.);
#6518=ORIENTED_EDGE('',*,*,#4822,.T.);
#6519=ORIENTED_EDGE('',*,*,#4818,.F.);
#6520=ORIENTED_EDGE('',*,*,#4822,.F.);
#6521=ORIENTED_EDGE('',*,*,#4823,.F.);
#6522=ORIENTED_EDGE('',*,*,#4824,.T.);
#6523=ORIENTED_EDGE('',*,*,#4825,.F.);
#6524=ORIENTED_EDGE('',*,*,#4824,.F.);
#6525=ORIENTED_EDGE('',*,*,#4826,.F.);
#6526=ORIENTED_EDGE('',*,*,#4827,.T.);
#6527=ORIENTED_EDGE('',*,*,#4828,.F.);
#6528=ORIENTED_EDGE('',*,*,#4827,.F.);
#6529=ORIENTED_EDGE('',*,*,#4829,.F.);
#6530=ORIENTED_EDGE('',*,*,#4830,.T.);
#6531=ORIENTED_EDGE('',*,*,#4819,.F.);
#6532=ORIENTED_EDGE('',*,*,#4830,.F.);
#6533=ORIENTED_EDGE('',*,*,#4831,.F.);
#6534=ORIENTED_EDGE('',*,*,#4832,.T.);
#6535=ORIENTED_EDGE('',*,*,#4833,.T.);
#6536=ORIENTED_EDGE('',*,*,#4832,.F.);
#6537=ORIENTED_EDGE('',*,*,#4833,.F.);
#6538=ORIENTED_EDGE('',*,*,#4834,.F.);
#6539=ORIENTED_EDGE('',*,*,#4835,.F.);
#6540=ORIENTED_EDGE('',*,*,#4836,.T.);
#6541=ORIENTED_EDGE('',*,*,#4837,.T.);
#6542=ORIENTED_EDGE('',*,*,#4836,.F.);
#6543=ORIENTED_EDGE('',*,*,#4837,.F.);
#6544=ORIENTED_EDGE('',*,*,#4838,.F.);
#6545=ORIENTED_EDGE('',*,*,#4834,.T.);
#6546=ORIENTED_EDGE('',*,*,#4839,.T.);
#6547=ORIENTED_EDGE('',*,*,#4840,.F.);
#6548=ORIENTED_EDGE('',*,*,#4839,.F.);
#6549=ORIENTED_EDGE('',*,*,#4838,.T.);
#6550=ORIENTED_EDGE('',*,*,#4841,.T.);
#6551=ORIENTED_EDGE('',*,*,#4842,.F.);
#6552=ORIENTED_EDGE('',*,*,#4841,.F.);
#6553=ORIENTED_EDGE('',*,*,#4843,.F.);
#6554=ORIENTED_EDGE('',*,*,#4844,.F.);
#6555=ORIENTED_EDGE('',*,*,#4845,.F.);
#6556=ORIENTED_EDGE('',*,*,#4846,.T.);
#6557=ORIENTED_EDGE('',*,*,#4847,.F.);
#6558=ORIENTED_EDGE('',*,*,#4848,.T.);
#6559=ORIENTED_EDGE('',*,*,#4849,.F.);
#6560=ORIENTED_EDGE('',*,*,#4850,.F.);
#6561=ORIENTED_EDGE('',*,*,#4851,.F.);
#6562=ORIENTED_EDGE('',*,*,#4852,.T.);
#6563=ORIENTED_EDGE('',*,*,#4853,.F.);
#6564=ORIENTED_EDGE('',*,*,#4854,.F.);
#6565=ORIENTED_EDGE('',*,*,#4855,.F.);
#6566=ORIENTED_EDGE('',*,*,#4856,.T.);
#6567=ORIENTED_EDGE('',*,*,#4857,.F.);
#6568=ORIENTED_EDGE('',*,*,#4858,.F.);
#6569=ORIENTED_EDGE('',*,*,#4859,.F.);
#6570=ORIENTED_EDGE('',*,*,#4860,.T.);
#6571=ORIENTED_EDGE('',*,*,#4861,.F.);
#6572=ORIENTED_EDGE('',*,*,#4862,.F.);
#6573=ORIENTED_EDGE('',*,*,#4863,.F.);
#6574=ORIENTED_EDGE('',*,*,#4864,.F.);
#6575=ORIENTED_EDGE('',*,*,#4865,.F.);
#6576=ORIENTED_EDGE('',*,*,#4866,.T.);
#6577=ORIENTED_EDGE('',*,*,#4867,.F.);
#6578=ORIENTED_EDGE('',*,*,#4868,.F.);
#6579=ORIENTED_EDGE('',*,*,#4869,.F.);
#6580=ORIENTED_EDGE('',*,*,#4870,.T.);
#6581=ORIENTED_EDGE('',*,*,#4871,.F.);
#6582=ORIENTED_EDGE('',*,*,#4840,.T.);
#6583=ORIENTED_EDGE('',*,*,#4872,.F.);
#6584=ORIENTED_EDGE('',*,*,#4842,.T.);
#6585=ORIENTED_EDGE('',*,*,#4873,.F.);
#6586=ORIENTED_EDGE('',*,*,#4846,.F.);
#6587=ORIENTED_EDGE('',*,*,#4874,.F.);
#6588=ORIENTED_EDGE('',*,*,#4860,.F.);
#6589=ORIENTED_EDGE('',*,*,#4875,.F.);
#6590=ORIENTED_EDGE('',*,*,#4866,.F.);
#6591=ORIENTED_EDGE('',*,*,#4876,.F.);
#6592=ORIENTED_EDGE('',*,*,#4848,.F.);
#6593=ORIENTED_EDGE('',*,*,#4877,.F.);
#6594=ORIENTED_EDGE('',*,*,#4870,.F.);
#6595=ORIENTED_EDGE('',*,*,#4878,.F.);
#6596=ORIENTED_EDGE('',*,*,#4852,.F.);
#6597=ORIENTED_EDGE('',*,*,#4879,.F.);
#6598=ORIENTED_EDGE('',*,*,#4880,.F.);
#6599=ORIENTED_EDGE('',*,*,#4881,.F.);
#6600=ORIENTED_EDGE('',*,*,#4856,.F.);
#6601=ORIENTED_EDGE('',*,*,#4882,.F.);
#6602=ORIENTED_EDGE('',*,*,#4883,.F.);
#6603=ORIENTED_EDGE('',*,*,#4884,.F.);
#6604=ORIENTED_EDGE('',*,*,#4880,.T.);
#6605=ORIENTED_EDGE('',*,*,#4885,.T.);
#6606=ORIENTED_EDGE('',*,*,#4886,.F.);
#6607=ORIENTED_EDGE('',*,*,#4887,.F.);
#6608=ORIENTED_EDGE('',*,*,#4816,.F.);
#6609=ORIENTED_EDGE('',*,*,#4812,.F.);
#6610=ORIENTED_EDGE('',*,*,#4888,.F.);
#6611=ORIENTED_EDGE('',*,*,#4857,.T.);
#6612=ORIENTED_EDGE('',*,*,#4881,.T.);
#6613=ORIENTED_EDGE('',*,*,#4884,.T.);
#6614=ORIENTED_EDGE('',*,*,#4889,.T.);
#6615=ORIENTED_EDGE('',*,*,#4890,.F.);
#6616=ORIENTED_EDGE('',*,*,#4810,.F.);
#6617=ORIENTED_EDGE('',*,*,#4815,.F.);
#6618=ORIENTED_EDGE('',*,*,#4891,.F.);
#6619=ORIENTED_EDGE('',*,*,#4892,.F.);
#6620=ORIENTED_EDGE('',*,*,#4893,.T.);
#6621=ORIENTED_EDGE('',*,*,#4853,.T.);
#6622=ORIENTED_EDGE('',*,*,#4878,.T.);
#6623=ORIENTED_EDGE('',*,*,#4869,.T.);
#6624=ORIENTED_EDGE('',*,*,#4894,.T.);
#6625=ORIENTED_EDGE('',*,*,#4895,.F.);
#6626=ORIENTED_EDGE('',*,*,#4896,.F.);
#6627=ORIENTED_EDGE('',*,*,#4897,.F.);
#6628=ORIENTED_EDGE('',*,*,#4898,.F.);
#6629=ORIENTED_EDGE('',*,*,#4899,.F.);
#6630=ORIENTED_EDGE('',*,*,#4900,.T.);
#6631=ORIENTED_EDGE('',*,*,#4849,.T.);
#6632=ORIENTED_EDGE('',*,*,#4876,.T.);
#6633=ORIENTED_EDGE('',*,*,#4865,.T.);
#6634=ORIENTED_EDGE('',*,*,#4901,.T.);
#6635=ORIENTED_EDGE('',*,*,#4902,.F.);
#6636=ORIENTED_EDGE('',*,*,#4805,.F.);
#6637=ORIENTED_EDGE('',*,*,#4903,.F.);
#6638=ORIENTED_EDGE('',*,*,#4904,.F.);
#6639=ORIENTED_EDGE('',*,*,#4905,.F.);
#6640=ORIENTED_EDGE('',*,*,#4906,.T.);
#6641=ORIENTED_EDGE('',*,*,#4843,.T.);
#6642=ORIENTED_EDGE('',*,*,#4873,.T.);
#6643=ORIENTED_EDGE('',*,*,#4859,.T.);
#6644=ORIENTED_EDGE('',*,*,#4907,.F.);
#6645=ORIENTED_EDGE('',*,*,#4908,.T.);
#6646=ORIENTED_EDGE('',*,*,#4909,.T.);
#6647=ORIENTED_EDGE('',*,*,#4910,.T.);
#6648=ORIENTED_EDGE('',*,*,#4911,.F.);
#6649=ORIENTED_EDGE('',*,*,#4858,.T.);
#6650=ORIENTED_EDGE('',*,*,#4893,.F.);
#6651=ORIENTED_EDGE('',*,*,#4912,.T.);
#6652=ORIENTED_EDGE('',*,*,#4885,.F.);
#6653=ORIENTED_EDGE('',*,*,#4913,.T.);
#6654=ORIENTED_EDGE('',*,*,#4889,.F.);
#6655=ORIENTED_EDGE('',*,*,#4883,.T.);
#6656=ORIENTED_EDGE('',*,*,#4914,.F.);
#6657=ORIENTED_EDGE('',*,*,#4915,.T.);
#6658=ORIENTED_EDGE('',*,*,#4894,.F.);
#6659=ORIENTED_EDGE('',*,*,#4868,.T.);
#6660=ORIENTED_EDGE('',*,*,#4916,.F.);
#6661=ORIENTED_EDGE('',*,*,#4917,.T.);
#6662=ORIENTED_EDGE('',*,*,#4901,.F.);
#6663=ORIENTED_EDGE('',*,*,#4864,.T.);
#6664=ORIENTED_EDGE('',*,*,#4918,.F.);
#6665=ORIENTED_EDGE('',*,*,#4919,.T.);
#6666=ORIENTED_EDGE('',*,*,#4920,.T.);
#6667=ORIENTED_EDGE('',*,*,#4907,.T.);
#6668=ORIENTED_EDGE('',*,*,#4862,.T.);
#6669=ORIENTED_EDGE('',*,*,#4921,.T.);
#6670=ORIENTED_EDGE('',*,*,#4922,.F.);
#6671=ORIENTED_EDGE('',*,*,#4923,.T.);
#6672=ORIENTED_EDGE('',*,*,#4924,.F.);
#6673=ORIENTED_EDGE('',*,*,#4925,.T.);
#6674=ORIENTED_EDGE('',*,*,#4926,.F.);
#6675=ORIENTED_EDGE('',*,*,#4927,.T.);
#6676=ORIENTED_EDGE('',*,*,#4928,.F.);
#6677=ORIENTED_EDGE('',*,*,#4929,.T.);
#6678=ORIENTED_EDGE('',*,*,#4844,.T.);
#6679=ORIENTED_EDGE('',*,*,#4911,.T.);
#6680=ORIENTED_EDGE('',*,*,#4930,.T.);
#6681=ORIENTED_EDGE('',*,*,#4931,.T.);
#6682=ORIENTED_EDGE('',*,*,#4932,.F.);
#6683=ORIENTED_EDGE('',*,*,#4850,.T.);
#6684=ORIENTED_EDGE('',*,*,#4906,.F.);
#6685=ORIENTED_EDGE('',*,*,#4933,.T.);
#6686=ORIENTED_EDGE('',*,*,#4934,.F.);
#6687=ORIENTED_EDGE('',*,*,#4854,.T.);
#6688=ORIENTED_EDGE('',*,*,#4900,.F.);
#6689=ORIENTED_EDGE('',*,*,#4935,.T.);
#6690=ORIENTED_EDGE('',*,*,#4936,.F.);
#6691=ORIENTED_EDGE('',*,*,#4937,.T.);
#6692=ORIENTED_EDGE('',*,*,#4938,.T.);
#6693=ORIENTED_EDGE('',*,*,#4939,.T.);
#6694=ORIENTED_EDGE('',*,*,#4940,.T.);
#6695=ORIENTED_EDGE('',*,*,#4941,.T.);
#6696=ORIENTED_EDGE('',*,*,#4942,.F.);
#6697=ORIENTED_EDGE('',*,*,#4820,.F.);
#6698=ORIENTED_EDGE('',*,*,#4943,.T.);
#6699=ORIENTED_EDGE('',*,*,#4872,.T.);
#6700=ORIENTED_EDGE('',*,*,#4943,.F.);
#6701=ORIENTED_EDGE('',*,*,#4944,.F.);
#6702=ORIENTED_EDGE('',*,*,#4945,.T.);
#6703=ORIENTED_EDGE('',*,*,#4871,.T.);
#6704=ORIENTED_EDGE('',*,*,#4945,.F.);
#6705=ORIENTED_EDGE('',*,*,#4946,.F.);
#6706=ORIENTED_EDGE('',*,*,#4942,.T.);
#6707=ORIENTED_EDGE('',*,*,#4947,.F.);
#6708=ORIENTED_EDGE('',*,*,#4948,.F.);
#6709=ORIENTED_EDGE('',*,*,#4949,.F.);
#6710=ORIENTED_EDGE('',*,*,#4950,.F.);
#6711=ORIENTED_EDGE('',*,*,#4886,.T.);
#6712=ORIENTED_EDGE('',*,*,#4912,.F.);
#6713=ORIENTED_EDGE('',*,*,#4892,.T.);
#6714=ORIENTED_EDGE('',*,*,#4951,.T.);
#6715=ORIENTED_EDGE('',*,*,#4946,.T.);
#6716=ORIENTED_EDGE('',*,*,#4952,.T.);
#6717=ORIENTED_EDGE('',*,*,#4953,.T.);
#6718=ORIENTED_EDGE('',*,*,#4937,.F.);
#6719=ORIENTED_EDGE('',*,*,#4796,.T.);
#6720=ORIENTED_EDGE('',*,*,#4817,.F.);
#6721=ORIENTED_EDGE('',*,*,#4887,.T.);
#6722=ORIENTED_EDGE('',*,*,#4951,.F.);
#6723=ORIENTED_EDGE('',*,*,#4891,.T.);
#6724=ORIENTED_EDGE('',*,*,#4814,.F.);
#6725=ORIENTED_EDGE('',*,*,#4950,.T.);
#6726=ORIENTED_EDGE('',*,*,#4954,.F.);
#6727=ORIENTED_EDGE('',*,*,#4955,.F.);
#6728=ORIENTED_EDGE('',*,*,#4952,.F.);
#6729=ORIENTED_EDGE('',*,*,#4949,.T.);
#6730=ORIENTED_EDGE('',*,*,#4956,.T.);
#6731=ORIENTED_EDGE('',*,*,#4957,.T.);
#6732=ORIENTED_EDGE('',*,*,#4954,.T.);
#6733=ORIENTED_EDGE('',*,*,#4888,.T.);
#6734=ORIENTED_EDGE('',*,*,#4811,.T.);
#6735=ORIENTED_EDGE('',*,*,#4890,.T.);
#6736=ORIENTED_EDGE('',*,*,#4913,.F.);
#6737=ORIENTED_EDGE('',*,*,#4947,.T.);
#6738=ORIENTED_EDGE('',*,*,#4941,.F.);
#6739=ORIENTED_EDGE('',*,*,#4958,.T.);
#6740=ORIENTED_EDGE('',*,*,#4959,.T.);
#6741=ORIENTED_EDGE('',*,*,#4855,.T.);
#6742=ORIENTED_EDGE('',*,*,#4936,.T.);
#6743=ORIENTED_EDGE('',*,*,#4960,.F.);
#6744=ORIENTED_EDGE('',*,*,#4961,.F.);
#6745=ORIENTED_EDGE('',*,*,#4962,.F.);
#6746=ORIENTED_EDGE('',*,*,#4963,.F.);
#6747=ORIENTED_EDGE('',*,*,#4964,.F.);
#6748=ORIENTED_EDGE('',*,*,#4914,.T.);
#6749=ORIENTED_EDGE('',*,*,#4882,.T.);
#6750=ORIENTED_EDGE('',*,*,#4879,.T.);
#6751=ORIENTED_EDGE('',*,*,#4960,.T.);
#6752=ORIENTED_EDGE('',*,*,#4935,.F.);
#6753=ORIENTED_EDGE('',*,*,#4899,.T.);
#6754=ORIENTED_EDGE('',*,*,#4965,.T.);
#6755=ORIENTED_EDGE('',*,*,#4961,.T.);
#6756=ORIENTED_EDGE('',*,*,#4965,.F.);
#6757=ORIENTED_EDGE('',*,*,#4898,.T.);
#6758=ORIENTED_EDGE('',*,*,#4966,.F.);
#6759=ORIENTED_EDGE('',*,*,#4962,.T.);
#6760=ORIENTED_EDGE('',*,*,#4966,.T.);
#6761=ORIENTED_EDGE('',*,*,#4897,.T.);
#6762=ORIENTED_EDGE('',*,*,#4967,.T.);
#6763=ORIENTED_EDGE('',*,*,#4963,.T.);
#6764=ORIENTED_EDGE('',*,*,#4967,.F.);
#6765=ORIENTED_EDGE('',*,*,#4896,.T.);
#6766=ORIENTED_EDGE('',*,*,#4968,.F.);
#6767=ORIENTED_EDGE('',*,*,#4964,.T.);
#6768=ORIENTED_EDGE('',*,*,#4968,.T.);
#6769=ORIENTED_EDGE('',*,*,#4895,.T.);
#6770=ORIENTED_EDGE('',*,*,#4915,.F.);
#6771=ORIENTED_EDGE('',*,*,#4851,.T.);
#6772=ORIENTED_EDGE('',*,*,#4934,.T.);
#6773=ORIENTED_EDGE('',*,*,#4969,.F.);
#6774=ORIENTED_EDGE('',*,*,#4970,.F.);
#6775=ORIENTED_EDGE('',*,*,#4971,.F.);
#6776=ORIENTED_EDGE('',*,*,#4807,.F.);
#6777=ORIENTED_EDGE('',*,*,#4972,.F.);
#6778=ORIENTED_EDGE('',*,*,#4916,.T.);
#6779=ORIENTED_EDGE('',*,*,#4867,.T.);
#6780=ORIENTED_EDGE('',*,*,#4877,.T.);
#6781=ORIENTED_EDGE('',*,*,#4969,.T.);
#6782=ORIENTED_EDGE('',*,*,#4933,.F.);
#6783=ORIENTED_EDGE('',*,*,#4905,.T.);
#6784=ORIENTED_EDGE('',*,*,#4973,.T.);
#6785=ORIENTED_EDGE('',*,*,#4800,.T.);
#6786=ORIENTED_EDGE('',*,*,#4974,.F.);
#6787=ORIENTED_EDGE('',*,*,#4970,.T.);
#6788=ORIENTED_EDGE('',*,*,#4973,.F.);
#6789=ORIENTED_EDGE('',*,*,#4904,.T.);
#6790=ORIENTED_EDGE('',*,*,#4975,.F.);
#6791=ORIENTED_EDGE('',*,*,#4808,.T.);
#6792=ORIENTED_EDGE('',*,*,#4971,.T.);
#6793=ORIENTED_EDGE('',*,*,#4974,.T.);
#6794=ORIENTED_EDGE('',*,*,#4801,.F.);
#6795=ORIENTED_EDGE('',*,*,#4975,.T.);
#6796=ORIENTED_EDGE('',*,*,#4903,.T.);
#6797=ORIENTED_EDGE('',*,*,#4804,.T.);
#6798=ORIENTED_EDGE('',*,*,#4799,.F.);
#6799=ORIENTED_EDGE('',*,*,#4828,.T.);
#6800=ORIENTED_EDGE('',*,*,#4825,.T.);
#6801=ORIENTED_EDGE('',*,*,#4944,.T.);
#6802=ORIENTED_EDGE('',*,*,#4972,.T.);
#6803=ORIENTED_EDGE('',*,*,#4806,.T.);
#6804=ORIENTED_EDGE('',*,*,#4902,.T.);
#6805=ORIENTED_EDGE('',*,*,#4917,.F.);
#6806=ORIENTED_EDGE('',*,*,#4847,.T.);
#6807=ORIENTED_EDGE('',*,*,#4932,.T.);
#6808=ORIENTED_EDGE('',*,*,#4976,.F.);
#6809=ORIENTED_EDGE('',*,*,#4977,.F.);
#6810=ORIENTED_EDGE('',*,*,#4978,.F.);
#6811=ORIENTED_EDGE('',*,*,#4979,.F.);
#6812=ORIENTED_EDGE('',*,*,#4980,.F.);
#6813=ORIENTED_EDGE('',*,*,#4918,.T.);
#6814=ORIENTED_EDGE('',*,*,#4863,.T.);
#6815=ORIENTED_EDGE('',*,*,#4875,.T.);
#6816=ORIENTED_EDGE('',*,*,#4976,.T.);
#6817=ORIENTED_EDGE('',*,*,#4931,.F.);
#6818=ORIENTED_EDGE('',*,*,#4981,.T.);
#6819=ORIENTED_EDGE('',*,*,#4982,.T.);
#6820=ORIENTED_EDGE('',*,*,#4977,.T.);
#6821=ORIENTED_EDGE('',*,*,#4982,.F.);
#6822=ORIENTED_EDGE('',*,*,#4983,.F.);
#6823=ORIENTED_EDGE('',*,*,#4984,.F.);
#6824=ORIENTED_EDGE('',*,*,#4978,.T.);
#6825=ORIENTED_EDGE('',*,*,#4984,.T.);
#6826=ORIENTED_EDGE('',*,*,#4985,.T.);
#6827=ORIENTED_EDGE('',*,*,#4986,.T.);
#6828=ORIENTED_EDGE('',*,*,#4980,.T.);
#6829=ORIENTED_EDGE('',*,*,#4987,.T.);
#6830=ORIENTED_EDGE('',*,*,#4988,.T.);
#6831=ORIENTED_EDGE('',*,*,#4919,.F.);
#6832=ORIENTED_EDGE('',*,*,#4979,.T.);
#6833=ORIENTED_EDGE('',*,*,#4986,.F.);
#6834=ORIENTED_EDGE('',*,*,#4989,.F.);
#6835=ORIENTED_EDGE('',*,*,#4987,.F.);
#6836=ORIENTED_EDGE('',*,*,#4990,.T.);
#6837=ORIENTED_EDGE('',*,*,#4991,.T.);
#6838=ORIENTED_EDGE('',*,*,#4989,.T.);
#6839=ORIENTED_EDGE('',*,*,#4992,.T.);
#6840=ORIENTED_EDGE('',*,*,#4993,.T.);
#6841=ORIENTED_EDGE('',*,*,#4994,.T.);
#6842=ORIENTED_EDGE('',*,*,#4983,.T.);
#6843=ORIENTED_EDGE('',*,*,#4995,.T.);
#6844=ORIENTED_EDGE('',*,*,#4996,.T.);
#6845=ORIENTED_EDGE('',*,*,#4990,.F.);
#6846=ORIENTED_EDGE('',*,*,#4985,.F.);
#6847=ORIENTED_EDGE('',*,*,#4996,.F.);
#6848=ORIENTED_EDGE('',*,*,#4909,.F.);
#6849=ORIENTED_EDGE('',*,*,#4930,.F.);
#6850=ORIENTED_EDGE('',*,*,#4910,.F.);
#6851=ORIENTED_EDGE('',*,*,#4995,.F.);
#6852=ORIENTED_EDGE('',*,*,#4981,.F.);
#6853=ORIENTED_EDGE('',*,*,#4997,.T.);
#6854=ORIENTED_EDGE('',*,*,#4955,.T.);
#6855=ORIENTED_EDGE('',*,*,#4998,.T.);
#6856=ORIENTED_EDGE('',*,*,#4998,.F.);
#6857=ORIENTED_EDGE('',*,*,#4957,.F.);
#6858=ORIENTED_EDGE('',*,*,#4994,.F.);
#6859=ORIENTED_EDGE('',*,*,#4999,.F.);
#6860=ORIENTED_EDGE('',*,*,#4938,.F.);
#6861=ORIENTED_EDGE('',*,*,#4953,.F.);
#6862=ORIENTED_EDGE('',*,*,#4997,.F.);
#6863=ORIENTED_EDGE('',*,*,#5000,.F.);
#6864=ORIENTED_EDGE('',*,*,#4940,.F.);
#6865=ORIENTED_EDGE('',*,*,#5001,.F.);
#6866=ORIENTED_EDGE('',*,*,#4993,.F.);
#6867=ORIENTED_EDGE('',*,*,#4958,.F.);
#6868=ORIENTED_EDGE('',*,*,#4948,.T.);
#6869=ORIENTED_EDGE('',*,*,#4959,.F.);
#6870=ORIENTED_EDGE('',*,*,#4992,.F.);
#6871=ORIENTED_EDGE('',*,*,#4956,.F.);
#6872=ORIENTED_EDGE('',*,*,#4920,.F.);
#6873=ORIENTED_EDGE('',*,*,#4988,.F.);
#6874=ORIENTED_EDGE('',*,*,#4991,.F.);
#6875=ORIENTED_EDGE('',*,*,#4908,.F.);
#6876=ORIENTED_EDGE('',*,*,#5000,.T.);
#6877=ORIENTED_EDGE('',*,*,#4999,.T.);
#6878=ORIENTED_EDGE('',*,*,#5001,.T.);
#6879=ORIENTED_EDGE('',*,*,#4939,.F.);
#6880=ORIENTED_EDGE('',*,*,#5002,.F.);
#6881=ORIENTED_EDGE('',*,*,#5003,.F.);
#6882=ORIENTED_EDGE('',*,*,#5004,.F.);
#6883=ORIENTED_EDGE('',*,*,#5005,.F.);
#6884=ORIENTED_EDGE('',*,*,#5006,.F.);
#6885=ORIENTED_EDGE('',*,*,#5007,.F.);
#6886=ORIENTED_EDGE('',*,*,#5008,.F.);
#6887=ORIENTED_EDGE('',*,*,#5009,.F.);
#6888=ORIENTED_EDGE('',*,*,#5010,.F.);
#6889=ORIENTED_EDGE('',*,*,#5002,.T.);
#6890=ORIENTED_EDGE('',*,*,#5011,.T.);
#6891=ORIENTED_EDGE('',*,*,#5009,.T.);
#6892=ORIENTED_EDGE('',*,*,#5012,.T.);
#6893=ORIENTED_EDGE('',*,*,#4928,.T.);
#6894=ORIENTED_EDGE('',*,*,#5013,.T.);
#6895=ORIENTED_EDGE('',*,*,#5010,.T.);
#6896=ORIENTED_EDGE('',*,*,#5014,.T.);
#6897=ORIENTED_EDGE('',*,*,#5015,.F.);
#6898=ORIENTED_EDGE('',*,*,#5016,.F.);
#6899=ORIENTED_EDGE('',*,*,#5017,.F.);
#6900=ORIENTED_EDGE('',*,*,#5016,.T.);
#6901=ORIENTED_EDGE('',*,*,#5018,.T.);
#6902=ORIENTED_EDGE('',*,*,#5006,.T.);
#6903=ORIENTED_EDGE('',*,*,#5019,.T.);
#6904=ORIENTED_EDGE('',*,*,#5008,.T.);
#6905=ORIENTED_EDGE('',*,*,#5020,.T.);
#6906=ORIENTED_EDGE('',*,*,#5017,.T.);
#6907=ORIENTED_EDGE('',*,*,#5021,.T.);
#6908=ORIENTED_EDGE('',*,*,#4926,.T.);
#6909=ORIENTED_EDGE('',*,*,#5022,.T.);
#6910=ORIENTED_EDGE('',*,*,#5015,.T.);
#6911=ORIENTED_EDGE('',*,*,#5023,.T.);
#6912=ORIENTED_EDGE('',*,*,#4924,.T.);
#6913=ORIENTED_EDGE('',*,*,#5024,.T.);
#6914=ORIENTED_EDGE('',*,*,#5007,.T.);
#6915=ORIENTED_EDGE('',*,*,#5025,.T.);
#6916=ORIENTED_EDGE('',*,*,#5005,.T.);
#6917=ORIENTED_EDGE('',*,*,#5026,.T.);
#6918=ORIENTED_EDGE('',*,*,#5003,.T.);
#6919=ORIENTED_EDGE('',*,*,#5027,.T.);
#6920=ORIENTED_EDGE('',*,*,#4922,.T.);
#6921=ORIENTED_EDGE('',*,*,#5028,.T.);
#6922=ORIENTED_EDGE('',*,*,#5004,.T.);
#6923=ORIENTED_EDGE('',*,*,#5029,.T.);
#6924=ORIENTED_EDGE('',*,*,#5023,.F.);
#6925=ORIENTED_EDGE('',*,*,#5020,.F.);
#6926=ORIENTED_EDGE('',*,*,#5013,.F.);
#6927=ORIENTED_EDGE('',*,*,#4927,.F.);
#6928=ORIENTED_EDGE('',*,*,#4845,.T.);
#6929=ORIENTED_EDGE('',*,*,#4929,.F.);
#6930=ORIENTED_EDGE('',*,*,#5014,.F.);
#6931=ORIENTED_EDGE('',*,*,#5011,.F.);
#6932=ORIENTED_EDGE('',*,*,#5028,.F.);
#6933=ORIENTED_EDGE('',*,*,#4921,.F.);
#6934=ORIENTED_EDGE('',*,*,#4861,.T.);
#6935=ORIENTED_EDGE('',*,*,#4874,.T.);
#6936=ORIENTED_EDGE('',*,*,#5019,.F.);
#6937=ORIENTED_EDGE('',*,*,#5027,.F.);
#6938=ORIENTED_EDGE('',*,*,#5012,.F.);
#6939=ORIENTED_EDGE('',*,*,#5021,.F.);
#6940=ORIENTED_EDGE('',*,*,#4835,.T.);
#6941=ORIENTED_EDGE('',*,*,#4831,.T.);
#6942=ORIENTED_EDGE('',*,*,#4829,.T.);
#6943=ORIENTED_EDGE('',*,*,#4826,.T.);
#6944=ORIENTED_EDGE('',*,*,#4823,.T.);
#6945=ORIENTED_EDGE('',*,*,#4821,.T.);
#6946=ORIENTED_EDGE('',*,*,#5024,.F.);
#6947=ORIENTED_EDGE('',*,*,#4923,.F.);
#6948=ORIENTED_EDGE('',*,*,#5029,.F.);
#6949=ORIENTED_EDGE('',*,*,#5026,.F.);
#6950=ORIENTED_EDGE('',*,*,#5022,.F.);
#6951=ORIENTED_EDGE('',*,*,#4925,.F.);
#6952=ORIENTED_EDGE('',*,*,#5025,.F.);
#6953=ORIENTED_EDGE('',*,*,#5018,.F.);
#8197=CYLINDRICAL_SURFACE('',#9089,0.25);
#8198=CYLINDRICAL_SURFACE('',#9091,0.25);
#8199=CYLINDRICAL_SURFACE('',#9093,0.25);
#8200=CYLINDRICAL_SURFACE('',#9095,0.25);
#8201=CYLINDRICAL_SURFACE('',#9101,0.15);
#8202=CYLINDRICAL_SURFACE('',#9103,0.15);
#8203=CYLINDRICAL_SURFACE('',#9106,0.15);
#8204=CYLINDRICAL_SURFACE('',#9109,0.15);
#8205=CYLINDRICAL_SURFACE('',#9111,0.3);
#8206=CYLINDRICAL_SURFACE('',#9116,0.3);
#8207=CYLINDRICAL_SURFACE('',#9121,0.17);
#8208=CYLINDRICAL_SURFACE('',#9123,0.17);
#8209=CYLINDRICAL_SURFACE('',#9147,0.4);
#8210=CYLINDRICAL_SURFACE('',#9148,0.4);
#8211=CYLINDRICAL_SURFACE('',#9171,0.1);
#8212=CYLINDRICAL_SURFACE('',#9175,0.1);
#8213=CYLINDRICAL_SURFACE('',#9189,0.3);
#8214=CYLINDRICAL_SURFACE('',#9194,0.3);
#8469=ADVANCED_FACE('',(#1052),#8197,.F.);
#8470=ADVANCED_FACE('',(#1053),#8198,.F.);
#8471=ADVANCED_FACE('',(#1054),#8199,.F.);
#8472=ADVANCED_FACE('',(#1055),#8200,.F.);
#8473=ADVANCED_FACE('',(#1056),#92,.T.);
#8474=ADVANCED_FACE('',(#1057),#93,.T.);
#8475=ADVANCED_FACE('',(#1058,#599,#600,#601),#789,.F.);
#8476=ADVANCED_FACE('',(#1059),#8201,.F.);
#8477=ADVANCED_FACE('',(#1060),#8202,.F.);
#8478=ADVANCED_FACE('',(#1061),#8203,.F.);
#8479=ADVANCED_FACE('',(#1062),#8204,.F.);
#8480=ADVANCED_FACE('',(#1063),#8205,.F.);
#8481=ADVANCED_FACE('',(#1064,#602),#790,.F.);
#8482=ADVANCED_FACE('',(#1065),#8206,.F.);
#8483=ADVANCED_FACE('',(#1066,#603),#791,.F.);
#8484=ADVANCED_FACE('',(#1067),#8207,.F.);
#8485=ADVANCED_FACE('',(#1068),#8208,.F.);
#8486=ADVANCED_FACE('',(#1069),#792,.F.);
#8487=ADVANCED_FACE('',(#1070),#793,.F.);
#8488=ADVANCED_FACE('',(#1071),#794,.F.);
#8489=ADVANCED_FACE('',(#1072),#795,.F.);
#8490=ADVANCED_FACE('',(#1073),#796,.F.);
#8491=ADVANCED_FACE('',(#1074),#797,.F.);
#8492=ADVANCED_FACE('',(#1075),#798,.F.);
#8493=ADVANCED_FACE('',(#1076,#604),#799,.F.);
#8494=ADVANCED_FACE('',(#1077,#605),#800,.F.);
#8495=ADVANCED_FACE('',(#1078),#801,.F.);
#8496=ADVANCED_FACE('',(#1079),#802,.F.);
#8497=ADVANCED_FACE('',(#1080),#803,.F.);
#8498=ADVANCED_FACE('',(#1081),#804,.F.);
#8499=ADVANCED_FACE('',(#1082),#805,.F.);
#8500=ADVANCED_FACE('',(#1083),#806,.T.);
#8501=ADVANCED_FACE('',(#1084),#807,.T.);
#8502=ADVANCED_FACE('',(#1085),#808,.T.);
#8503=ADVANCED_FACE('',(#1086),#809,.T.);
#8504=ADVANCED_FACE('',(#1087),#810,.T.);
#8505=ADVANCED_FACE('',(#1088,#606),#811,.F.);
#8506=ADVANCED_FACE('',(#1089),#8209,.T.);
#8507=ADVANCED_FACE('',(#1090),#8210,.T.);
#8508=ADVANCED_FACE('',(#1091),#812,.T.);
#8509=ADVANCED_FACE('',(#1092),#94,.T.);
#8510=ADVANCED_FACE('',(#1093),#95,.T.);
#8511=ADVANCED_FACE('',(#1094),#96,.T.);
#8512=ADVANCED_FACE('',(#1095),#97,.T.);
#8513=ADVANCED_FACE('',(#1096),#813,.F.);
#8514=ADVANCED_FACE('',(#1097),#98,.T.);
#8515=ADVANCED_FACE('',(#1098),#99,.T.);
#8516=ADVANCED_FACE('',(#1099),#814,.T.);
#8517=ADVANCED_FACE('',(#1100),#100,.T.);
#8518=ADVANCED_FACE('',(#1101),#101,.T.);
#8519=ADVANCED_FACE('',(#1102),#815,.F.);
#8520=ADVANCED_FACE('',(#1103),#102,.T.);
#8521=ADVANCED_FACE('',(#1104),#103,.T.);
#8522=ADVANCED_FACE('',(#1105),#816,.T.);
#8523=ADVANCED_FACE('',(#1106),#104,.T.);
#8524=ADVANCED_FACE('',(#1107),#105,.T.);
#8525=ADVANCED_FACE('',(#1108,#607,#608,#609),#817,.F.);
#8526=ADVANCED_FACE('',(#1109),#106,.T.);
#8527=ADVANCED_FACE('',(#1110),#818,.T.);
#8528=ADVANCED_FACE('',(#1111),#107,.T.);
#8529=ADVANCED_FACE('',(#1112),#108,.T.);
#8530=ADVANCED_FACE('',(#1113),#819,.F.);
#8531=ADVANCED_FACE('',(#1114),#109,.T.);
#8532=ADVANCED_FACE('',(#1115),#110,.T.);
#8533=ADVANCED_FACE('',(#1116),#76,.F.);
#8534=ADVANCED_FACE('',(#1117),#77,.F.);
#8535=ADVANCED_FACE('',(#1118),#78,.F.);
#8536=ADVANCED_FACE('',(#1119),#8211,.F.);
#8537=ADVANCED_FACE('',(#1120),#111,.T.);
#8538=ADVANCED_FACE('',(#1121),#79,.F.);
#8539=ADVANCED_FACE('',(#1122),#8212,.F.);
#8540=ADVANCED_FACE('',(#1123),#112,.T.);
#8541=ADVANCED_FACE('',(#1124),#113,.T.);
#8542=ADVANCED_FACE('',(#1125),#114,.T.);
#8543=ADVANCED_FACE('',(#1126),#115,.T.);
#8544=ADVANCED_FACE('',(#1127),#820,.T.);
#8545=ADVANCED_FACE('',(#1128),#80,.T.);
#8546=ADVANCED_FACE('',(#1129),#81,.T.);
#8547=ADVANCED_FACE('',(#1130),#82,.T.);
#8548=ADVANCED_FACE('',(#1131),#8213,.T.);
#8549=ADVANCED_FACE('',(#1132),#116,.F.);
#8550=ADVANCED_FACE('',(#1133),#83,.T.);
#8551=ADVANCED_FACE('',(#1134),#8214,.T.);
#8552=ADVANCED_FACE('',(#1135),#117,.F.);
#8553=ADVANCED_FACE('',(#1136),#118,.F.);
#8554=ADVANCED_FACE('',(#1137),#119,.F.);
#8555=ADVANCED_FACE('',(#1138),#120,.F.);
#8556=ADVANCED_FACE('',(#1139),#121,.F.);
#8557=ADVANCED_FACE('',(#1140),#122,.F.);
#8558=ADVANCED_FACE('',(#1141),#821,.F.);
#8559=ADVANCED_FACE('',(#1142,#610,#611,#612,#613,#614,#615),#822,.T.);
#8560=ADVANCED_FACE('',(#1143),#123,.F.);
#8561=ADVANCED_FACE('',(#1144),#823,.F.);
#8806=CLOSED_SHELL('',(#8469,#8470,#8471,#8472,#8473,#8474,#8475,#8476,
#8477,#8478,#8479,#8480,#8481,#8482,#8483,#8484,#8485,#8486,#8487,#8488,
#8489,#8490,#8491,#8492,#8493,#8494,#8495,#8496,#8497,#8498,#8499,#8500,
#8501,#8502,#8503,#8504,#8505,#8506,#8507,#8508,#8509,#8510,#8511,#8512,
#8513,#8514,#8515,#8516,#8517,#8518,#8519,#8520,#8521,#8522,#8523,#8524,
#8525,#8526,#8527,#8528,#8529,#8530,#8531,#8532,#8533,#8534,#8535,#8536,
#8537,#8538,#8539,#8540,#8541,#8542,#8543,#8544,#8545,#8546,#8547,#8548,
#8549,#8550,#8551,#8552,#8553,#8554,#8555,#8556,#8557,#8558,#8559,#8560,
#8561));
#9088=AXIS2_PLACEMENT_3D('',#12260,#10250,#10251);
#9089=AXIS2_PLACEMENT_3D('',#12261,#10252,#10253);
#9090=AXIS2_PLACEMENT_3D('',#12288,#10254,#10255);
#9091=AXIS2_PLACEMENT_3D('',#12289,#10256,#10257);
#9092=AXIS2_PLACEMENT_3D('',#12312,#10258,#10259);
#9093=AXIS2_PLACEMENT_3D('',#12313,#10260,#10261);
#9094=AXIS2_PLACEMENT_3D('',#12336,#10262,#10263);
#9095=AXIS2_PLACEMENT_3D('',#12337,#10264,#10265);
#9096=AXIS2_PLACEMENT_3D('',#12364,#10266,#10267);
#9097=AXIS2_PLACEMENT_3D('',#12549,#10268,#10269);
#9098=AXIS2_PLACEMENT_3D('',#12563,#10272,#10273);
#9099=AXIS2_PLACEMENT_3D('',#12565,#10274,#10275);
#9100=AXIS2_PLACEMENT_3D('',#12567,#10276,#10277);
#9101=AXIS2_PLACEMENT_3D('',#12568,#10278,#10279);
#9102=AXIS2_PLACEMENT_3D('',#12570,#10280,#10281);
#9103=AXIS2_PLACEMENT_3D('',#12572,#10283,#10284);
#9104=AXIS2_PLACEMENT_3D('',#12574,#10285,#10286);
#9105=AXIS2_PLACEMENT_3D('',#12577,#10288,#10289);
#9106=AXIS2_PLACEMENT_3D('',#12578,#10290,#10291);
#9107=AXIS2_PLACEMENT_3D('',#12580,#10292,#10293);
#9108=AXIS2_PLACEMENT_3D('',#12583,#10295,#10296);
#9109=AXIS2_PLACEMENT_3D('',#12584,#10297,#10298);
#9110=AXIS2_PLACEMENT_3D('',#12586,#10299,#10300);
#9111=AXIS2_PLACEMENT_3D('',#12588,#10302,#10303);
#9112=AXIS2_PLACEMENT_3D('',#12590,#10304,#10305);
#9113=AXIS2_PLACEMENT_3D('',#12593,#10307,#10308);
#9114=AXIS2_PLACEMENT_3D('',#12594,#10309,#10310);
#9115=AXIS2_PLACEMENT_3D('',#12596,#10311,#10312);
#9116=AXIS2_PLACEMENT_3D('',#12597,#10313,#10314);
#9117=AXIS2_PLACEMENT_3D('',#12599,#10315,#10316);
#9118=AXIS2_PLACEMENT_3D('',#12602,#10318,#10319);
#9119=AXIS2_PLACEMENT_3D('',#12603,#10320,#10321);
#9120=AXIS2_PLACEMENT_3D('',#12605,#10322,#10323);
#9121=AXIS2_PLACEMENT_3D('',#12606,#10324,#10325);
#9122=AXIS2_PLACEMENT_3D('',#12609,#10327,#10328);
#9123=AXIS2_PLACEMENT_3D('',#12610,#10329,#10330);
#9124=AXIS2_PLACEMENT_3D('',#12613,#10332,#10333);
#9125=AXIS2_PLACEMENT_3D('',#12614,#10334,#10335);
#9126=AXIS2_PLACEMENT_3D('',#12623,#10340,#10341);
#9127=AXIS2_PLACEMENT_3D('',#12632,#10346,#10347);
#9128=AXIS2_PLACEMENT_3D('',#12641,#10352,#10353);
#9129=AXIS2_PLACEMENT_3D('',#12650,#10358,#10359);
#9130=AXIS2_PLACEMENT_3D('',#12659,#10364,#10365);
#9131=AXIS2_PLACEMENT_3D('',#12668,#10370,#10371);
#9132=AXIS2_PLACEMENT_3D('',#12677,#10376,#10377);
#9133=AXIS2_PLACEMENT_3D('',#12679,#10378,#10379);
#9134=AXIS2_PLACEMENT_3D('',#12680,#10380,#10381);
#9135=AXIS2_PLACEMENT_3D('',#12682,#10382,#10383);
#9136=AXIS2_PLACEMENT_3D('',#12683,#10384,#10385);
#9137=AXIS2_PLACEMENT_3D('',#12686,#10388,#10389);
#9138=AXIS2_PLACEMENT_3D('',#12689,#10392,#10393);
#9139=AXIS2_PLACEMENT_3D('',#12692,#10396,#10397);
#9140=AXIS2_PLACEMENT_3D('',#12698,#10401,#10402);
#9141=AXIS2_PLACEMENT_3D('',#12704,#10406,#10407);
#9142=AXIS2_PLACEMENT_3D('',#12749,#10409,#10410);
#9143=AXIS2_PLACEMENT_3D('',#12795,#10413,#10414);
#9144=AXIS2_PLACEMENT_3D('',#12873,#10418,#10419);
#9145=AXIS2_PLACEMENT_3D('',#12921,#10423,#10424);
#9146=AXIS2_PLACEMENT_3D('',#12937,#10428,#10429);
#9147=AXIS2_PLACEMENT_3D('',#13258,#10441,#10442);
#9148=AXIS2_PLACEMENT_3D('',#13260,#10444,#10445);
#9149=AXIS2_PLACEMENT_3D('',#13262,#10446,#10447);
#9150=AXIS2_PLACEMENT_3D('',#13264,#10449,#10450);
#9151=AXIS2_PLACEMENT_3D('',#13428,#10452,#10453);
#9152=AXIS2_PLACEMENT_3D('',#13429,#10454,#10455);
#9153=AXIS2_PLACEMENT_3D('',#13477,#10457,#10458);
#9154=AXIS2_PLACEMENT_3D('',#13595,#10460,#10461);
#9155=AXIS2_PLACEMENT_3D('',#13640,#10462,#10463);
#9156=AXIS2_PLACEMENT_3D('',#13732,#10465,#10466);
#9157=AXIS2_PLACEMENT_3D('',#13749,#10467,#10468);
#9158=AXIS2_PLACEMENT_3D('',#13869,#10470,#10471);
#9159=AXIS2_PLACEMENT_3D('',#13874,#10472,#10473);
#9160=AXIS2_PLACEMENT_3D('',#13926,#10475,#10476);
#9161=AXIS2_PLACEMENT_3D('',#13927,#10477,#10478);
#9162=AXIS2_PLACEMENT_3D('',#13928,#10479,#10480);
#9163=AXIS2_PLACEMENT_3D('',#13929,#10481,#10482);
#9164=AXIS2_PLACEMENT_3D('',#13930,#10483,#10484);
#9165=AXIS2_PLACEMENT_3D('',#13931,#10485,#10486);
#9166=AXIS2_PLACEMENT_3D('',#13933,#10487,#10488);
#9167=AXIS2_PLACEMENT_3D('',#13934,#10489,#10490);
#9168=AXIS2_PLACEMENT_3D('',#13935,#10491,#10492);
#9169=AXIS2_PLACEMENT_3D('',#13936,#10493,#10494);
#9170=AXIS2_PLACEMENT_3D('',#13937,#10495,#10496);
#9171=AXIS2_PLACEMENT_3D('',#13938,#10497,#10498);
#9172=AXIS2_PLACEMENT_3D('',#13959,#10499,#10500);
#9173=AXIS2_PLACEMENT_3D('',#13961,#10501,#10502);
#9174=AXIS2_PLACEMENT_3D('',#13962,#10503,#10504);
#9175=AXIS2_PLACEMENT_3D('',#13963,#10505,#10506);
#9176=AXIS2_PLACEMENT_3D('',#14053,#10508,#10509);
#9177=AXIS2_PLACEMENT_3D('',#14054,#10510,#10511);
#9178=AXIS2_PLACEMENT_3D('',#14057,#10512,#10513);
#9179=AXIS2_PLACEMENT_3D('',#14059,#10514,#10515);
#9180=AXIS2_PLACEMENT_3D('',#14060,#10516,#10517);
#9181=AXIS2_PLACEMENT_3D('',#14061,#10518,#10519);
#9182=AXIS2_PLACEMENT_3D('',#14064,#10520,#10521);
#9183=AXIS2_PLACEMENT_3D('',#14066,#10522,#10523);
#9184=AXIS2_PLACEMENT_3D('',#14067,#10524,#10525);
#9185=AXIS2_PLACEMENT_3D('',#14068,#10526,#10527);
#9186=AXIS2_PLACEMENT_3D('',#14071,#10528,#10529);
#9187=AXIS2_PLACEMENT_3D('',#14073,#10530,#10531);
#9188=AXIS2_PLACEMENT_3D('',#14074,#10532,#10533);
#9189=AXIS2_PLACEMENT_3D('',#14075,#10534,#10535);
#9190=AXIS2_PLACEMENT_3D('',#14106,#10538,#10539);
#9191=AXIS2_PLACEMENT_3D('',#14109,#10540,#10541);
#9192=AXIS2_PLACEMENT_3D('',#14111,#10542,#10543);
#9193=AXIS2_PLACEMENT_3D('',#14112,#10544,#10545);
#9194=AXIS2_PLACEMENT_3D('',#14113,#10546,#10547);
#9195=AXIS2_PLACEMENT_3D('',#14286,#10550,#10551);
#9196=AXIS2_PLACEMENT_3D('',#14287,#10552,#10553);
#9197=AXIS2_PLACEMENT_3D('',#14304,#10554,#10555);
#10250=DIRECTION('axis',(0.,0.,1.));
#10251=DIRECTION('refdir',(1.,0.,0.));
#10252=DIRECTION('center_axis',(0.,0.,-1.));
#10253=DIRECTION('ref_axis',(1.,0.,0.));
#10254=DIRECTION('center_axis',(0.,0.,1.));
#10255=DIRECTION('ref_axis',(1.,0.,0.));
#10256=DIRECTION('center_axis',(0.,0.,-1.));
#10257=DIRECTION('ref_axis',(1.,0.,0.));
#10258=DIRECTION('center_axis',(0.,0.,1.));
#10259=DIRECTION('ref_axis',(1.,0.,0.));
#10260=DIRECTION('center_axis',(0.,0.,-1.));
#10261=DIRECTION('ref_axis',(1.,0.,0.));
#10262=DIRECTION('center_axis',(0.,0.,1.));
#10263=DIRECTION('ref_axis',(1.,0.,0.));
#10264=DIRECTION('center_axis',(0.,0.,-1.));
#10265=DIRECTION('ref_axis',(1.,0.,0.));
#10266=DIRECTION('center_axis',(0.,0.,1.));
#10267=DIRECTION('ref_axis',(1.,0.,0.));
#10268=DIRECTION('center_axis',(4.10828654779316E-33,-1.13946463231163E-19,
1.));
#10269=DIRECTION('ref_axis',(1.,0.,-4.10828654779316E-33));
#10270=DIRECTION('',(0.,1.,1.13946463231163E-19));
#10271=DIRECTION('',(0.,-1.,-1.13946463231163E-19));
#10272=DIRECTION('center_axis',(4.10828654779316E-33,-1.13946463231163E-19,
1.));
#10273=DIRECTION('ref_axis',(1.,0.,0.));
#10274=DIRECTION('center_axis',(4.10828654779316E-33,-1.13946463231163E-19,
1.));
#10275=DIRECTION('ref_axis',(1.,0.,0.));
#10276=DIRECTION('center_axis',(4.10828654779316E-33,-1.13946463231163E-19,
1.));
#10277=DIRECTION('ref_axis',(1.,0.,0.));
#10278=DIRECTION('center_axis',(0.,0.,-1.));
#10279=DIRECTION('ref_axis',(1.,0.,0.));
#10280=DIRECTION('center_axis',(-4.10828654779316E-33,1.13946463231163E-19,
-1.));
#10281=DIRECTION('ref_axis',(1.,0.,0.));
#10282=DIRECTION('',(0.,0.,-1.));
#10283=DIRECTION('center_axis',(0.,0.,-1.));
#10284=DIRECTION('ref_axis',(1.,0.,0.));
#10285=DIRECTION('center_axis',(-4.10828654779316E-33,1.13946463231163E-19,
-1.));
#10286=DIRECTION('ref_axis',(1.,0.,0.));
#10287=DIRECTION('',(0.,0.,-1.));
#10288=DIRECTION('center_axis',(4.10828654779316E-33,-1.13946463231163E-19,
1.));
#10289=DIRECTION('ref_axis',(1.,0.,0.));
#10290=DIRECTION('center_axis',(0.,0.,-1.));
#10291=DIRECTION('ref_axis',(1.,0.,0.));
#10292=DIRECTION('center_axis',(-4.10828654779316E-33,1.13946463231163E-19,
-1.));
#10293=DIRECTION('ref_axis',(1.,0.,0.));
#10294=DIRECTION('',(0.,0.,-1.));
#10295=DIRECTION('center_axis',(4.10828654779316E-33,-1.13946463231163E-19,
1.));
#10296=DIRECTION('ref_axis',(1.,0.,0.));
#10297=DIRECTION('center_axis',(0.,0.,-1.));
#10298=DIRECTION('ref_axis',(1.,0.,0.));
#10299=DIRECTION('center_axis',(-4.10828654779316E-33,1.13946463231163E-19,
-1.));
#10300=DIRECTION('ref_axis',(1.,0.,0.));
#10301=DIRECTION('',(0.,0.,-1.));
#10302=DIRECTION('center_axis',(0.,0.,-1.));
#10303=DIRECTION('ref_axis',(1.,0.,0.));
#10304=DIRECTION('center_axis',(-4.10828654779316E-33,1.13946463231163E-19,
-1.));
#10305=DIRECTION('ref_axis',(1.,0.,0.));
#10306=DIRECTION('',(0.,0.,-1.));
#10307=DIRECTION('center_axis',(0.,0.,-1.));
#10308=DIRECTION('ref_axis',(1.,0.,0.));
#10309=DIRECTION('center_axis',(0.,0.,-1.));
#10310=DIRECTION('ref_axis',(1.,0.,0.));
#10311=DIRECTION('center_axis',(0.,0.,1.));
#10312=DIRECTION('ref_axis',(1.,0.,0.));
#10313=DIRECTION('center_axis',(0.,0.,-1.));
#10314=DIRECTION('ref_axis',(1.,0.,0.));
#10315=DIRECTION('center_axis',(-4.10828654779316E-33,1.13946463231163E-19,
-1.));
#10316=DIRECTION('ref_axis',(1.,0.,0.));
#10317=DIRECTION('',(0.,0.,-1.));
#10318=DIRECTION('center_axis',(0.,0.,-1.));
#10319=DIRECTION('ref_axis',(1.,0.,0.));
#10320=DIRECTION('center_axis',(0.,0.,-1.));
#10321=DIRECTION('ref_axis',(1.,0.,0.));
#10322=DIRECTION('center_axis',(0.,0.,1.));
#10323=DIRECTION('ref_axis',(1.,0.,0.));
#10324=DIRECTION('center_axis',(0.,0.,-1.));
#10325=DIRECTION('ref_axis',(1.,0.,0.));
#10326=DIRECTION('',(0.,0.,-1.));
#10327=DIRECTION('center_axis',(0.,0.,1.));
#10328=DIRECTION('ref_axis',(1.,0.,0.));
#10329=DIRECTION('center_axis',(0.,0.,-1.));
#10330=DIRECTION('ref_axis',(1.,0.,0.));
#10331=DIRECTION('',(0.,0.,-1.));
#10332=DIRECTION('center_axis',(0.,0.,1.));
#10333=DIRECTION('ref_axis',(1.,0.,0.));
#10334=DIRECTION('center_axis',(0.,-1.,0.));
#10335=DIRECTION('ref_axis',(-1.,0.,0.));
#10336=DIRECTION('',(0.0523359562429438,0.,0.998629534754574));
#10337=DIRECTION('',(1.,0.,0.));
#10338=DIRECTION('',(-0.0523359562429438,0.,-0.998629534754574));
#10339=DIRECTION('',(1.,0.,0.));
#10340=DIRECTION('center_axis',(0.,-1.,0.));
#10341=DIRECTION('ref_axis',(-1.,0.,0.));
#10342=DIRECTION('',(0.,0.,-1.));
#10343=DIRECTION('',(1.,0.,0.));
#10344=DIRECTION('',(0.,0.,1.));
#10345=DIRECTION('',(1.,0.,0.));
#10346=DIRECTION('center_axis',(0.,-1.,0.));
#10347=DIRECTION('ref_axis',(-1.,0.,0.));
#10348=DIRECTION('',(0.,0.,-1.));
#10349=DIRECTION('',(1.,0.,0.));
#10350=DIRECTION('',(0.,0.,1.));
#10351=DIRECTION('',(1.,0.,0.));
#10352=DIRECTION('center_axis',(0.,-1.,0.));
#10353=DIRECTION('ref_axis',(-1.,0.,0.));
#10354=DIRECTION('',(0.,0.,-1.));
#10355=DIRECTION('',(1.,0.,0.));
#10356=DIRECTION('',(0.,0.,1.));
#10357=DIRECTION('',(1.,0.,0.));
#10358=DIRECTION('center_axis',(0.,1.,0.));
#10359=DIRECTION('ref_axis',(1.,0.,0.));
#10360=DIRECTION('',(-0.0523359562429438,0.,-0.998629534754574));
#10361=DIRECTION('',(-1.,0.,0.));
#10362=DIRECTION('',(0.0523359562429438,0.,0.998629534754574));
#10363=DIRECTION('',(-1.,0.,0.));
#10364=DIRECTION('center_axis',(0.,1.,0.));
#10365=DIRECTION('ref_axis',(1.,0.,0.));
#10366=DIRECTION('',(0.,0.,1.));
#10367=DIRECTION('',(-1.,0.,0.));
#10368=DIRECTION('',(0.,0.,-1.));
#10369=DIRECTION('',(-1.,0.,0.));
#10370=DIRECTION('center_axis',(0.,1.,0.));
#10371=DIRECTION('ref_axis',(1.,0.,0.));
#10372=DIRECTION('',(0.,0.,1.));
#10373=DIRECTION('',(-1.,0.,0.));
#10374=DIRECTION('',(0.,0.,-1.));
#10375=DIRECTION('',(-1.,0.,0.));
#10376=DIRECTION('center_axis',(0.,0.,1.));
#10377=DIRECTION('ref_axis',(1.,0.,0.));
#10378=DIRECTION('center_axis',(0.,0.,1.));
#10379=DIRECTION('ref_axis',(1.,0.,0.));
#10380=DIRECTION('center_axis',(0.,0.,1.));
#10381=DIRECTION('ref_axis',(1.,0.,0.));
#10382=DIRECTION('center_axis',(0.,0.,1.));
#10383=DIRECTION('ref_axis',(1.,0.,0.));
#10384=DIRECTION('center_axis',(0.,0.,1.));
#10385=DIRECTION('ref_axis',(1.,0.,0.));
#10386=DIRECTION('',(0.,1.,0.));
#10387=DIRECTION('',(0.,-1.,0.));
#10388=DIRECTION('center_axis',(0.,0.,1.));
#10389=DIRECTION('ref_axis',(1.,0.,0.));
#10390=DIRECTION('',(0.,-1.,0.));
#10391=DIRECTION('',(0.,1.,0.));
#10392=DIRECTION('center_axis',(0.,0.,1.));
#10393=DIRECTION('ref_axis',(1.,0.,0.));
#10394=DIRECTION('',(0.,-1.,0.));
#10395=DIRECTION('',(0.,1.,0.));
#10396=DIRECTION('center_axis',(0.,0.,1.));
#10397=DIRECTION('ref_axis',(1.,0.,0.));
#10398=DIRECTION('',(0.,-1.,0.));
#10399=DIRECTION('',(-1.,0.,0.));
#10400=DIRECTION('',(0.,1.,0.));
#10401=DIRECTION('center_axis',(0.,1.,0.));
#10402=DIRECTION('ref_axis',(1.,0.,0.));
#10403=DIRECTION('',(0.,0.,1.));
#10404=DIRECTION('',(-1.,0.,0.));
#10405=DIRECTION('',(0.,0.,-1.));
#10406=DIRECTION('center_axis',(-1.,0.,0.));
#10407=DIRECTION('ref_axis',(0.,-1.,0.));
#10408=DIRECTION('',(0.,-1.,0.));
#10409=DIRECTION('center_axis',(1.,0.,0.));
#10410=DIRECTION('ref_axis',(0.,1.,0.));
#10411=DIRECTION('',(0.,1.,0.));
#10412=DIRECTION('',(0.,1.,0.));
#10413=DIRECTION('center_axis',(1.,0.,0.));
#10414=DIRECTION('ref_axis',(0.,1.,0.));
#10415=DIRECTION('',(0.,1.,0.));
#10416=DIRECTION('',(0.,1.,1.13946463231163E-19));
#10417=DIRECTION('',(0.,1.,0.));
#10418=DIRECTION('center_axis',(1.,0.,0.));
#10419=DIRECTION('ref_axis',(0.,1.,0.));
#10420=DIRECTION('',(0.,1.,0.));
#10421=DIRECTION('',(0.,1.,1.13946463231163E-19));
#10422=DIRECTION('',(0.,1.,0.));
#10423=DIRECTION('center_axis',(0.998629534754574,0.,-0.0523359562429438));
#10424=DIRECTION('ref_axis',(-0.0523359562429438,0.,-0.998629534754574));
#10425=DIRECTION('',(0.,-1.,0.));
#10426=DIRECTION('',(-5.97168109510197E-21,-1.,-1.13946463231163E-19));
#10427=DIRECTION('',(0.,-1.,0.));
#10428=DIRECTION('center_axis',(0.,0.,1.));
#10429=DIRECTION('ref_axis',(1.,0.,0.));
#10430=DIRECTION('',(0.,-1.,0.));
#10431=DIRECTION('',(0.,-1.,0.));
#10432=DIRECTION('',(0.,-1.,0.));
#10433=DIRECTION('',(0.,1.,0.));
#10434=DIRECTION('',(0.,-1.,0.));
#10435=DIRECTION('',(0.,1.,0.));
#10436=DIRECTION('',(0.,-1.,0.));
#10437=DIRECTION('',(0.,-1.,0.));
#10438=DIRECTION('',(0.,-1.,0.));
#10439=DIRECTION('',(0.,1.,0.));
#10440=DIRECTION('',(0.,1.,0.));
#10441=DIRECTION('center_axis',(0.,0.,1.));
#10442=DIRECTION('ref_axis',(1.,0.,0.));
#10443=DIRECTION('',(0.,0.,-1.));
#10444=DIRECTION('center_axis',(0.,0.,1.));
#10445=DIRECTION('ref_axis',(1.,0.,0.));
#10446=DIRECTION('center_axis',(4.10828654779316E-33,-1.13946463231163E-19,
1.));
#10447=DIRECTION('ref_axis',(1.,0.,0.));
#10448=DIRECTION('',(0.,0.,-1.));
#10449=DIRECTION('center_axis',(1.,0.,0.));
#10450=DIRECTION('ref_axis',(0.,1.,0.));
#10451=DIRECTION('',(0.,1.,1.13946463231163E-19));
#10452=DIRECTION('center_axis',(0.99852593895705,0.0542765992849681,9.38276897523041E-9));
#10453=DIRECTION('ref_axis',(0.0541946171271057,-0.99701772369063,0.0549418066794405));
#10454=DIRECTION('center_axis',(4.10828654779316E-33,-1.13946463231163E-19,
1.));
#10455=DIRECTION('ref_axis',(1.,0.,-4.10828654779316E-33));
#10456=DIRECTION('',(5.97168109510217E-21,-1.,-1.13946463231163E-19));
#10457=DIRECTION('center_axis',(-1.,0.,0.));
#10458=DIRECTION('ref_axis',(0.,-1.,0.));
#10459=DIRECTION('',(0.,-1.,-1.13946463231163E-19));
#10460=DIRECTION('center_axis',(4.10828654779316E-33,-1.13946463231163E-19,
1.));
#10461=DIRECTION('ref_axis',(1.,0.,-4.10828654779316E-33));
#10462=DIRECTION('center_axis',(-1.,0.,0.));
#10463=DIRECTION('ref_axis',(0.,-1.,0.));
#10464=DIRECTION('',(0.,-1.,-1.13946463231163E-19));
#10465=DIRECTION('center_axis',(4.10828654779316E-33,-1.13946463231163E-19,
1.));
#10466=DIRECTION('ref_axis',(1.,0.,-4.10828654779316E-33));
#10467=DIRECTION('center_axis',(-1.,0.,0.));
#10468=DIRECTION('ref_axis',(0.,-1.,0.));
#10469=DIRECTION('',(0.,-1.,-1.13946463231163E-19));
#10470=DIRECTION('center_axis',(-0.996961060527779,0.0779015005717205,0.));
#10471=DIRECTION('ref_axis',(0.,0.,1.));
#10472=DIRECTION('center_axis',(4.10828654779316E-33,-1.13946463231163E-19,
1.));
#10473=DIRECTION('ref_axis',(1.,0.,-4.10828654779316E-33));
#10474=DIRECTION('',(5.97168109510197E-21,1.,1.13946463231163E-19));
#10475=DIRECTION('center_axis',(-0.996961060527779,-0.0779015005717276,
-4.485055189269E-15));
#10476=DIRECTION('ref_axis',(-0.0777791112471086,0.995394757055134,0.0560329142626144));
#10477=DIRECTION('center_axis',(-0.377317868652411,-0.840644185582845,0.388521015186253));
#10478=DIRECTION('ref_axis',(-0.58566693710526,0.541587807512093,0.603056287203763));
#10479=DIRECTION('center_axis',(7.41164423166535E-16,1.,0.));
#10480=DIRECTION('ref_axis',(0.,0.,1.));
#10481=DIRECTION('center_axis',(0.0522650005536027,-0.0520548592672972,
0.997275619547472));
#10482=DIRECTION('ref_axis',(-0.998629534754574,7.40148683083438E-16,0.0523359562429445));
#10483=DIRECTION('center_axis',(0.376559988603802,-0.837471124372148,0.396036224133039));
#10484=DIRECTION('ref_axis',(0.577069986161316,0.546481578685729,0.606916893181374));
#10485=DIRECTION('center_axis',(0.998525938475037,-0.0542766081525538,0.));
#10486=DIRECTION('ref_axis',(0.,0.,1.));
#10487=DIRECTION('center_axis',(-0.0522648366634829,-0.0521149007022807,
0.997272492337641));
#10488=DIRECTION('ref_axis',(0.0541946171271058,0.99701772369063,0.0549418066794413));
#10489=DIRECTION('center_axis',(5.32220538281047E-11,1.,-1.01553728389566E-9));
#10490=DIRECTION('ref_axis',(0.998629534754574,0.,0.0523359562429456));
#10491=DIRECTION('center_axis',(0.37731786865241,-0.840644185582843,-0.388521015186259));
#10492=DIRECTION('ref_axis',(-0.585666937105255,-0.541587807512095,0.603056287203766));
#10493=DIRECTION('center_axis',(0.0522650005536027,0.0520548592672965,0.997275619547472));
#10494=DIRECTION('ref_axis',(-0.0777791112471059,-0.995394757055134,0.0560329142626137));
#10495=DIRECTION('center_axis',(0.,-1.,0.));
#10496=DIRECTION('ref_axis',(-0.998629534754574,0.,0.0523359562429439));
#10497=DIRECTION('center_axis',(5.97168109510197E-21,1.,1.13946463231163E-19));
#10498=DIRECTION('ref_axis',(-0.688354575693753,0.,0.725374371012288));
#10499=DIRECTION('center_axis',(-0.376559987018669,-0.837471124206646,-0.396036225990193));
#10500=DIRECTION('ref_axis',(0.577069983350267,-0.54648157893936,0.606916895625808));
#10501=DIRECTION('center_axis',(-0.0522648366634817,0.0521149007022785,
0.997272492337641));
#10502=DIRECTION('ref_axis',(0.998629534754574,0.,0.052335956242946));
#10503=DIRECTION('center_axis',(1.01693095242295E-9,-1.,0.));
#10504=DIRECTION('ref_axis',(0.,0.,1.));
#10505=DIRECTION('center_axis',(5.97168109510217E-21,-1.,-1.13946463231163E-19));
#10506=DIRECTION('ref_axis',(0.688354575693753,0.,0.725374371012289));
#10507=DIRECTION('',(-5.97168109510217E-21,1.,1.13946463231163E-19));
#10508=DIRECTION('center_axis',(-0.998629534754574,0.,-0.0523359562429455));
#10509=DIRECTION('ref_axis',(-0.0523359562429455,0.,0.998629534754574));
#10510=DIRECTION('center_axis',(-0.377317868652411,-0.840644185582845,0.388521015186254));
#10511=DIRECTION('ref_axis',(-0.585666937105261,0.541587807512092,0.603056287203763));
#10512=DIRECTION('center_axis',(7.41164423166535E-16,1.,0.));
#10513=DIRECTION('ref_axis',(0.,0.,1.));
#10514=DIRECTION('center_axis',(-0.996961060527779,-0.0779015005717276,
-4.485055189269E-15));
#10515=DIRECTION('ref_axis',(-0.0777791112471086,0.995394757055134,0.0560329142626144));
#10516=DIRECTION('center_axis',(0.0522650005536027,-0.0520548592672972,
0.997275619547472));
#10517=DIRECTION('ref_axis',(-0.998629534754574,7.40148683083438E-16,0.0523359562429445));
#10518=DIRECTION('center_axis',(0.376559988603802,-0.837471124372148,0.396036224133039));
#10519=DIRECTION('ref_axis',(0.577069986161311,0.546481578685732,0.606916893181376));
#10520=DIRECTION('center_axis',(0.998525938475037,-0.0542766081525538,0.));
#10521=DIRECTION('ref_axis',(0.,0.,1.));
#10522=DIRECTION('center_axis',(5.32220538281047E-11,1.,-1.01553728389566E-9));
#10523=DIRECTION('ref_axis',(0.998629534754574,0.,0.0523359562429456));
#10524=DIRECTION('center_axis',(-0.0522648366634829,-0.0521149007022807,
0.997272492337641));
#10525=DIRECTION('ref_axis',(0.0541946171271058,0.99701772369063,0.0549418066794413));
#10526=DIRECTION('center_axis',(0.37731786865241,-0.840644185582843,-0.388521015186259));
#10527=DIRECTION('ref_axis',(-0.585666937105255,-0.541587807512095,0.603056287203766));
#10528=DIRECTION('center_axis',(-0.996961060527779,0.0779015005717205,0.));
#10529=DIRECTION('ref_axis',(0.,0.,1.));
#10530=DIRECTION('center_axis',(0.,-1.,0.));
#10531=DIRECTION('ref_axis',(-0.998629534754574,0.,0.0523359562429439));
#10532=DIRECTION('center_axis',(0.0522650005536027,0.0520548592672965,0.997275619547472));
#10533=DIRECTION('ref_axis',(-0.0777791112471059,-0.995394757055134,0.0560329142626137));
#10534=DIRECTION('center_axis',(5.97168109510197E-21,1.,1.13946463231163E-19));
#10535=DIRECTION('ref_axis',(-0.688354575693753,0.,0.725374371012289));
#10536=DIRECTION('',(-5.97168109510197E-21,-1.,-1.13946463231163E-19));
#10537=DIRECTION('',(5.97168109510197E-21,1.,1.13946463231163E-19));
#10538=DIRECTION('center_axis',(-0.376559987018669,-0.837471124206646,-0.396036225990194));
#10539=DIRECTION('ref_axis',(0.577069983350267,-0.546481578939359,0.606916895625808));
#10540=DIRECTION('center_axis',(-0.0522648366634817,0.0521149007022785,
0.997272492337641));
#10541=DIRECTION('ref_axis',(0.998629534754574,0.,0.052335956242946));
#10542=DIRECTION('center_axis',(1.01693095242295E-9,-1.,0.));
#10543=DIRECTION('ref_axis',(0.,0.,1.));
#10544=DIRECTION('center_axis',(0.99852593895705,0.0542765992849681,9.38276897523041E-9));
#10545=DIRECTION('ref_axis',(0.0541946171271057,-0.99701772369063,0.0549418066794405));
#10546=DIRECTION('center_axis',(5.97168109510217E-21,-1.,-1.13946463231163E-19));
#10547=DIRECTION('ref_axis',(0.688354575693753,0.,0.725374371012289));
#10548=DIRECTION('',(-5.97168109510217E-21,1.,1.13946463231163E-19));
#10549=DIRECTION('',(5.97168109510217E-21,-1.,-1.13946463231163E-19));
#10550=DIRECTION('center_axis',(0.998629534754574,0.,-0.0523359562429438));
#10551=DIRECTION('ref_axis',(-0.0523359562429438,0.,-0.998629534754574));
#10552=DIRECTION('center_axis',(4.10828654779316E-33,-1.13946463231163E-19,
1.));
#10553=DIRECTION('ref_axis',(1.,0.,-4.10828654779316E-33));
#10554=DIRECTION('center_axis',(-0.998629534754574,0.,-0.0523359562429455));
#10555=DIRECTION('ref_axis',(-0.0523359562429455,0.,0.998629534754574));
#12260=CARTESIAN_POINT('',(0.,0.,0.));
#12261=CARTESIAN_POINT('Origin',(8.1,-1.,0.7));
#12262=CARTESIAN_POINT('',(7.94916965151797,-1.19937453693185,0.7));
#12263=CARTESIAN_POINT('',(8.26514540988519,-1.18768855477586,0.7));
#12264=CARTESIAN_POINT('Ctrl Pts',(7.94916965151797,-1.19937453693185,0.7));
#12265=CARTESIAN_POINT('Ctrl Pts',(7.97160858810976,-1.21634998764782,0.7));
#12266=CARTESIAN_POINT('Ctrl Pts',(7.99739856866269,-1.22989011121344,0.69528529300377));
#12267=CARTESIAN_POINT('Ctrl Pts',(8.03944443766207,-1.24298414277179,0.688517705185315));
#12268=CARTESIAN_POINT('Ctrl Pts',(8.05362924383607,-1.24609346022897,0.686388676887586));
#12269=CARTESIAN_POINT('Ctrl Pts',(8.075506183533,-1.24890990228851,0.684139035126277));
#12270=CARTESIAN_POINT('Ctrl Pts',(8.08297567221474,-1.24953307703463,0.683546226354886));
#12271=CARTESIAN_POINT('Ctrl Pts',(8.0940066533036,-1.24995288972095,0.68299521602547));
#12272=CARTESIAN_POINT('Ctrl Pts',(8.09752287926269,-1.25001251279495,0.68286729538075));
#12273=CARTESIAN_POINT('Ctrl Pts',(8.10293413375911,-1.249989933108,0.682747340264197));
#12274=CARTESIAN_POINT('Ctrl Pts',(8.10482478940148,-1.24996059450444,0.682719828470948));
#12275=CARTESIAN_POINT('Ctrl Pts',(8.10828546792054,-1.24986760009171,0.682696100760705));
#12276=CARTESIAN_POINT('Ctrl Pts',(8.10985478687837,-1.24981062779486,0.682695370268813));
#12277=CARTESIAN_POINT('Ctrl Pts',(8.11326464342549,-1.24965465239671,0.682715595753076));
#12278=CARTESIAN_POINT('Ctrl Pts',(8.11510409202247,-1.2495501177419,0.682740330911594));
#12279=CARTESIAN_POINT('Ctrl Pts',(8.12014207260669,-1.24920790966494,0.682845651127781));
#12280=CARTESIAN_POINT('Ctrl Pts',(8.12333423895876,-1.24892926854386,0.682953992816581));
#12281=CARTESIAN_POINT('Ctrl Pts',(8.139194120874,-1.2472372768871,0.683691668462565));
#12282=CARTESIAN_POINT('Ctrl Pts',(8.15164141295685,-1.2449338270761,0.684918799511701));
#12283=CARTESIAN_POINT('Ctrl Pts',(8.19196937649467,-1.23428099896052,0.690212518998986));
#12284=CARTESIAN_POINT('Ctrl Pts',(8.21811504697062,-1.22213176592155,0.695755006185672));
#12285=CARTESIAN_POINT('Ctrl Pts',(8.24962874265135,-1.20052913769617,0.699397421419897));
#12286=CARTESIAN_POINT('Ctrl Pts',(8.25758631484639,-1.19433973204149,0.7));
#12287=CARTESIAN_POINT('Ctrl Pts',(8.26514540988519,-1.18768855477586,0.7));
#12288=CARTESIAN_POINT('Origin',(8.1,-1.,0.7));
#12289=CARTESIAN_POINT('Origin',(2.7,1.,0.7));
#12290=CARTESIAN_POINT('',(2.8076286513348,1.22564590451442,0.7));
#12291=CARTESIAN_POINT('',(2.57739843082973,1.21787348447435,0.7));
#12292=CARTESIAN_POINT('Ctrl Pts',(2.80762864495888,1.22564590575571,0.7));
#12293=CARTESIAN_POINT('Ctrl Pts',(2.78743249310418,1.23527907171202,0.7));
#12294=CARTESIAN_POINT('Ctrl Pts',(2.76507271635938,1.24261561512899,0.698430289974852));
#12295=CARTESIAN_POINT('Ctrl Pts',(2.73219941643314,1.24807722603274,0.696876198609429));
#12296=CARTESIAN_POINT('Ctrl Pts',(2.72335305886828,1.24906618730719,0.696525251810408));
#12297=CARTESIAN_POINT('Ctrl Pts',(2.71018695034311,1.24982905432238,0.696188910804419));
#12298=CARTESIAN_POINT('Ctrl Pts',(2.70590779780308,1.24996687586326,0.696107915309552));
#12299=CARTESIAN_POINT('Ctrl Pts',(2.69921702211412,1.25001037316246,0.696030339680738));
#12300=CARTESIAN_POINT('Ctrl Pts',(2.69680890442544,1.24999123464332,0.696012302673685));
#12301=CARTESIAN_POINT('Ctrl Pts',(2.69234597975348,1.24989125947742,0.695997601992606));
#12302=CARTESIAN_POINT('Ctrl Pts',(2.69029169500035,1.24981988388707,0.69599819279703));
#12303=CARTESIAN_POINT('Ctrl Pts',(2.6857660481318,1.24960673159635,0.696015705561832));
#12304=CARTESIAN_POINT('Ctrl Pts',(2.68329599580702,1.24945360531346,0.696035938105249));
#12305=CARTESIAN_POINT('Ctrl Pts',(2.67625328071593,1.24891193026541,0.696123377063474));
#12306=CARTESIAN_POINT('Ctrl Pts',(2.67169109188753,1.24843439216159,0.696216059649547));
#12307=CARTESIAN_POINT('Ctrl Pts',(2.64765560351845,1.24524789167778,0.696873729305584));
#12308=CARTESIAN_POINT('Ctrl Pts',(2.62857598726268,1.24037162800668,0.698048768812303));
#12309=CARTESIAN_POINT('Ctrl Pts',(2.59902076831046,1.22902239593109,0.699541037747764));
#12310=CARTESIAN_POINT('Ctrl Pts',(2.58799157881597,1.22383445108162,0.7));
#12311=CARTESIAN_POINT('Ctrl Pts',(2.57739843082979,1.21787348447436,0.7));
#12312=CARTESIAN_POINT('Origin',(2.7,1.,0.7));
#12313=CARTESIAN_POINT('Origin',(2.7,-1.,0.7));
#12314=CARTESIAN_POINT('',(2.57739843082979,-1.21787348447436,0.7));
#12315=CARTESIAN_POINT('',(2.80762864495888,-1.22564590575571,0.7));
#12316=CARTESIAN_POINT('Ctrl Pts',(2.57739843082979,-1.21787348447436,0.7));
#12317=CARTESIAN_POINT('Ctrl Pts',(2.59689796709118,-1.22884624579732,0.7));
#12318=CARTESIAN_POINT('Ctrl Pts',(2.61871070177046,-1.23767364961455,0.698430520021629));
#12319=CARTESIAN_POINT('Ctrl Pts',(2.6511387549791,-1.24533993869645,0.696876447160353));
#12320=CARTESIAN_POINT('Ctrl Pts',(2.65989793055836,-1.24692336726652,0.696525471319567));
#12321=CARTESIAN_POINT('Ctrl Pts',(2.67298219502323,-1.24857266139659,0.696189053183015));
#12322=CARTESIAN_POINT('Ctrl Pts',(2.67724223626036,-1.24899884484677,0.696108027479433));
#12323=CARTESIAN_POINT('Ctrl Pts',(2.68391475503581,-1.24949361628703,0.696030400846995));
#12324=CARTESIAN_POINT('Ctrl Pts',(2.68631866330158,-1.24963697932539,0.69601234479389));
#12325=CARTESIAN_POINT('Ctrl Pts',(2.69077815115796,-1.24983831390468,0.695997608323079));
#12326=CARTESIAN_POINT('Ctrl Pts',(2.69283257145917,-1.24990568929416,0.695998182544699));
#12327=CARTESIAN_POINT('Ctrl Pts',(2.69736230434386,-1.24999833696454,0.696015659042177));
#12328=CARTESIAN_POINT('Ctrl Pts',(2.69983707579759,-1.25001219669429,0.696035872086962));
#12329=CARTESIAN_POINT('Ctrl Pts',(2.70690037992806,-1.24994687665095,0.696123257636812));
#12330=CARTESIAN_POINT('Ctrl Pts',(2.71148446565418,-1.24977820005943,0.696215908504701));
#12331=CARTESIAN_POINT('Ctrl Pts',(2.73568105999059,-1.24822038288304,0.696873447340259));
#12332=CARTESIAN_POINT('Ctrl Pts',(2.75504695022812,-1.24464213141243,0.698048515307351));
#12333=CARTESIAN_POINT('Ctrl Pts',(2.78530198112344,-1.2353118289445,0.699540950501024));
#12334=CARTESIAN_POINT('Ctrl Pts',(2.79665680001786,-1.23087925931356,0.7));
#12335=CARTESIAN_POINT('Ctrl Pts',(2.80762864495888,-1.22564590575571,0.7));
#12336=CARTESIAN_POINT('Origin',(2.7,-1.,0.7));
#12337=CARTESIAN_POINT('Origin',(8.1,1.,0.7));
#12338=CARTESIAN_POINT('',(8.26514540988519,1.18768855477586,0.7));
#12339=CARTESIAN_POINT('',(7.94916965249954,1.19937453719419,0.7));
#12340=CARTESIAN_POINT('Ctrl Pts',(8.26514540988519,1.18768855477586,0.7));
#12341=CARTESIAN_POINT('Ctrl Pts',(8.24402114884725,1.20627559516199,0.7));
#12342=CARTESIAN_POINT('Ctrl Pts',(8.21930102059268,1.22168408824046,0.695284768760077));
#12343=CARTESIAN_POINT('Ctrl Pts',(8.17833936508797,1.23784683595578,0.688517484674842));
#12344=CARTESIAN_POINT('Ctrl Pts',(8.16442627443898,1.24199461640617,0.686388979601913));
#12345=CARTESIAN_POINT('Ctrl Pts',(8.14282164862934,1.24641910835203,0.684139556285851));
#12346=CARTESIAN_POINT('Ctrl Pts',(8.13541969045672,1.24759243465272,0.683546718614312));
#12347=CARTESIAN_POINT('Ctrl Pts',(8.12445132655127,1.24882623938238,0.682995554842566));
#12348=CARTESIAN_POINT('Ctrl Pts',(8.12094947916695,1.24914555886372,0.68286756899844));
#12349=CARTESIAN_POINT('Ctrl Pts',(8.11555178799172,1.24952297970176,0.682747494033431));
#12350=CARTESIAN_POINT('Ctrl Pts',(8.11366421100955,1.24963346420394,0.682719937279798));
#12351=CARTESIAN_POINT('Ctrl Pts',(8.11020620287515,1.24979651712922,0.682696124556263));
#12352=CARTESIAN_POINT('Ctrl Pts',(8.10863696767328,1.24985569708818,0.682695355189016));
#12353=CARTESIAN_POINT('Ctrl Pts',(8.10522484403353,1.249952190393,0.682715496638402));
#12354=CARTESIAN_POINT('Ctrl Pts',(8.10338263267786,1.24998390529834,0.682740187713169));
#12355=CARTESIAN_POINT('Ctrl Pts',(8.09833277498968,1.25001501472208,0.682845394223802));
#12356=CARTESIAN_POINT('Ctrl Pts',(8.09512844909059,1.24997307323179,0.682953673497893));
#12357=CARTESIAN_POINT('Ctrl Pts',(8.07918314804204,1.24945780552822,0.683691186949858));
#12358=CARTESIAN_POINT('Ctrl Pts',(8.06659630270856,1.24808001426183,0.684918585227095));
#12359=CARTESIAN_POINT('Ctrl Pts',(8.02558960427868,1.24043495378573,0.69021260546313));
#12360=CARTESIAN_POINT('Ctrl Pts',(7.9986188553413,1.2302509517108,0.695754623970086));
#12361=CARTESIAN_POINT('Ctrl Pts',(7.96559475436581,1.21103543221342,0.69939729083119));
#12362=CARTESIAN_POINT('Ctrl Pts',(7.95720051358587,1.20545002552208,0.7));
#12363=CARTESIAN_POINT('Ctrl Pts',(7.94916965151797,1.19937453693185,0.7));
#12364=CARTESIAN_POINT('Origin',(8.1,1.,0.7));
#12365=CARTESIAN_POINT('Ctrl Pts',(1.1,1.14549341399196,0.7));
#12366=CARTESIAN_POINT('Ctrl Pts',(1.89984199608574,1.1957170361627,0.7));
#12367=CARTESIAN_POINT('Ctrl Pts',(2.70080437300401,1.2273695200909,0.7));
#12368=CARTESIAN_POINT('Ctrl Pts',(3.50204003610941,1.24374118183538,0.7));
#12369=CARTESIAN_POINT('Ctrl Pts',(1.09819048660397,1.17431102498992,0.7));
#12370=CARTESIAN_POINT('Ctrl Pts',(1.89847848223077,1.22458382597074,0.70000077422621));
#12371=CARTESIAN_POINT('Ctrl Pts',(2.69984520196781,1.25626413437997,0.699999727319846));
#12372=CARTESIAN_POINT('Ctrl Pts',(3.50144932661635,1.27265074030048,0.700000000000001));
#12373=CARTESIAN_POINT('Ctrl Pts',(1.09505363188407,1.22426736091617,0.676703190608825));
#12374=CARTESIAN_POINT('Ctrl Pts',(1.89610976425884,1.27462253270773,0.67666760713801));
#12375=CARTESIAN_POINT('Ctrl Pts',(2.69818680938115,1.3063522351595,0.67664530655333));
#12376=CARTESIAN_POINT('Ctrl Pts',(3.50042536655637,1.322763754511,0.676632802377821));
#12377=CARTESIAN_POINT('Ctrl Pts',(1.09381704710221,1.24396073223232,0.627109609335854));
#12378=CARTESIAN_POINT('Ctrl Pts',(1.89518106151152,1.29430885982199,0.62701751976321));
#12379=CARTESIAN_POINT('Ctrl Pts',(2.69753328610131,1.32603127467068,0.626959208652505));
#12380=CARTESIAN_POINT('Ctrl Pts',(3.50002334924346,1.34243864233338,0.626926882269943));
#12381=CARTESIAN_POINT('Ctrl Pts',(1.09374258853658,1.24514653057163,0.605486452199395));
#12382=CARTESIAN_POINT('Ctrl Pts',(1.89512529323683,1.29547288309274,0.605377720397184));
#12383=CARTESIAN_POINT('Ctrl Pts',(2.69749615303001,1.32718177535833,0.605308474776761));
#12384=CARTESIAN_POINT('Ctrl Pts',(3.5,1.34358136363184,0.605270327458635));
#12385=CARTESIAN_POINT('',(1.1,1.14549341399195,0.7));
#12386=CARTESIAN_POINT('Ctrl Pts',(1.1,1.14549341399196,0.7));
#12387=CARTESIAN_POINT('Ctrl Pts',(1.59210562457523,1.17639367564078,0.7));
#12388=CARTESIAN_POINT('Ctrl Pts',(2.08463535466703,1.20026407570248,0.7));
#12389=CARTESIAN_POINT('Ctrl Pts',(2.57739190516306,1.2178709162388,0.7));
#12390=CARTESIAN_POINT('',(1.1,1.24553911298206,0.605485603995113));
#12391=CARTESIAN_POINT('Ctrl Pts',(1.1,1.14549341399196,0.7));
#12392=CARTESIAN_POINT('Ctrl Pts',(1.1,1.15341616150799,0.7));
#12393=CARTESIAN_POINT('Ctrl Pts',(1.1000012416168,1.16127613060545,0.699006361583129));
#12394=CARTESIAN_POINT('Ctrl Pts',(1.10000231308998,1.16893252943985,0.697119293189023));
#12395=CARTESIAN_POINT('Ctrl Pts',(1.10000291357081,1.17322337016277,0.696061732044743));
#12396=CARTESIAN_POINT('Ctrl Pts',(1.10000345673767,1.17745032641463,0.694722535963768));
#12397=CARTESIAN_POINT('Ctrl Pts',(1.10000379529503,1.18158693416151,0.693112479763539));
#12398=CARTESIAN_POINT('Ctrl Pts',(1.1000044034764,1.18901789868739,0.690220189452084));
#12399=CARTESIAN_POINT('Ctrl Pts',(1.1000042334852,1.19607766167095,0.686488065947256));
#12400=CARTESIAN_POINT('Ctrl Pts',(1.10000339376692,1.2026196529327,0.681996646156542));
#12401=CARTESIAN_POINT('Ctrl Pts',(1.10000293249552,1.20621327895058,0.67952943359521));
#12402=CARTESIAN_POINT('Ctrl Pts',(1.10000228571683,1.20965039763183,0.676832226278619));
#12403=CARTESIAN_POINT('Ctrl Pts',(1.10000171524363,1.21290279159005,0.673912896410569));
#12404=CARTESIAN_POINT('Ctrl Pts',(1.10000115816795,1.2160788033717,0.671062126739188));
#12405=CARTESIAN_POINT('Ctrl Pts',(1.10000066850715,1.2190594221245,0.668016750164662));
#12406=CARTESIAN_POINT('Ctrl Pts',(1.10000067525152,1.22182202639256,0.664788091882127));
#12407=CARTESIAN_POINT('Ctrl Pts',(1.10000068775799,1.22694487635592,0.658801012170571));
#12408=CARTESIAN_POINT('Ctrl Pts',(1.10000222199399,1.23132099043293,0.652185071179834));
#12409=CARTESIAN_POINT('Ctrl Pts',(1.10000276904041,1.23488987417606,0.64510534613808));
#12410=CARTESIAN_POINT('Ctrl Pts',(1.10000282439334,1.23525099193115,0.644388983656765));
#12411=CARTESIAN_POINT('Ctrl Pts',(1.10000287212626,1.23560380546488,0.64366785367332));
#12412=CARTESIAN_POINT('Ctrl Pts',(1.10000291138002,1.23594822450451,0.642942116631622));
#12413=CARTESIAN_POINT('Ctrl Pts',(1.10000329911404,1.23935026814133,0.635773555081239));
#12414=CARTESIAN_POINT('Ctrl Pts',(1.10000258010782,1.24189771450306,0.628240464257889));
#12415=CARTESIAN_POINT('Ctrl Pts',(1.10000149084855,1.24353681278199,0.620511076118615));
#12416=CARTESIAN_POINT('Ctrl Pts',(1.10000079446814,1.24458471384188,0.615569557890241));
#12417=CARTESIAN_POINT('Ctrl Pts',(1.10000000111128,1.24526049271905,0.610547146027233));
#12418=CARTESIAN_POINT('Ctrl Pts',(1.09999999916631,1.24553911263843,0.605485603997432));
#12419=CARTESIAN_POINT('',(3.5,1.34358136363184,0.605270327458635));
#12420=CARTESIAN_POINT('Ctrl Pts',(3.5,1.34358136363184,0.605270327458635));
#12421=CARTESIAN_POINT('Ctrl Pts',(2.6995848679345,1.32722445934619,0.605308375488923));
#12422=CARTESIAN_POINT('Ctrl Pts',(1.89930203168261,1.29563783986497,0.605377360150118));
#12423=CARTESIAN_POINT('Ctrl Pts',(1.09999999916631,1.24553911263843,0.605485603997431));
#12424=CARTESIAN_POINT('',(3.5,1.24369946473792,0.7));
#12425=CARTESIAN_POINT('Ctrl Pts',(3.5,1.34358136363184,0.605270327458635));
#12426=CARTESIAN_POINT('Ctrl Pts',(3.5,1.34316359984937,0.613184373088104));
#12427=CARTESIAN_POINT('Ctrl Pts',(3.50000057901142,1.34177887744868,0.621008021569537));
#12428=CARTESIAN_POINT('Ctrl Pts',(3.50000082863025,1.33951086762262,0.628580534231506));
#12429=CARTESIAN_POINT('Ctrl Pts',(3.50000096811,1.33824356956914,0.632811834486987));
#12430=CARTESIAN_POINT('Ctrl Pts',(3.50000102536574,1.33669948631919,0.636964759527324));
#12431=CARTESIAN_POINT('Ctrl Pts',(3.50000098105742,1.334886463945,0.641009258704104));
#12432=CARTESIAN_POINT('Ctrl Pts',(3.50000090179773,1.3316432906201,0.648244145614236));
#12433=CARTESIAN_POINT('Ctrl Pts',(3.50000044940971,1.3275777080273,0.655054131048541));
#12434=CARTESIAN_POINT('Ctrl Pts',(3.50000027423476,1.32275302640998,0.661275670751788));
#12435=CARTESIAN_POINT('Ctrl Pts',(3.50000024156065,1.32185311357394,0.66243612938574));
#12436=CARTESIAN_POINT('Ctrl Pts',(3.50000022115524,1.32092666334894,0.663576045687695));
#12437=CARTESIAN_POINT('Ctrl Pts',(3.50000022069074,1.31997391848392,0.664694242102532));
#12438=CARTESIAN_POINT('Ctrl Pts',(3.50000021976176,1.31806844339147,0.666930617752677));
#12439=CARTESIAN_POINT('Ctrl Pts',(3.50000029790302,1.31605782519,0.669080165434128));
#12440=CARTESIAN_POINT('Ctrl Pts',(3.50000040488465,1.31394946763378,0.671139079687271));
#12441=CARTESIAN_POINT('Ctrl Pts',(3.50000069329649,1.3082655455861,0.6766897075128));
#12442=CARTESIAN_POINT('Ctrl Pts',(3.5000011432336,1.30193818666762,0.681521899278667));
#12443=CARTESIAN_POINT('Ctrl Pts',(3.50000129797765,1.29513115062548,0.68558123547136));
#12444=CARTESIAN_POINT('Ctrl Pts',(3.50000139624096,1.2908086457691,0.688158936000333));
#12445=CARTESIAN_POINT('Ctrl Pts',(3.50000139493488,1.28629176508013,0.690424313967808));
#12446=CARTESIAN_POINT('Ctrl Pts',(3.50000129141552,1.28161680488022,0.692354162840695));
#12447=CARTESIAN_POINT('Ctrl Pts',(3.50000112941005,1.27430059661786,0.695374333209024));
#12448=CARTESIAN_POINT('Ctrl Pts',(3.5000007162179,1.26668229982361,0.697540280949125));
#12449=CARTESIAN_POINT('Ctrl Pts',(3.50000038344698,1.25890895215876,0.698782355543395));
#12450=CARTESIAN_POINT('Ctrl Pts',(3.50000016866387,1.25389173534334,0.699584038140014));
#12451=CARTESIAN_POINT('Ctrl Pts',(3.4999999993056,1.24880933504677,0.69999999987784));
#12452=CARTESIAN_POINT('Ctrl Pts',(3.49999999991873,1.24369946470729,0.7));
#12453=CARTESIAN_POINT('Ctrl Pts',(2.80762377174497,1.22564400643366,0.7));
#12454=CARTESIAN_POINT('Ctrl Pts',(3.03837960601223,1.23298334400942,0.7));
#12455=CARTESIAN_POINT('Ctrl Pts',(3.26917843294065,1.23897560812206,0.7));
#12456=CARTESIAN_POINT('Ctrl Pts',(3.49999999991873,1.24369946470729,0.7));
#12457=CARTESIAN_POINT('Ctrl Pts',(7.29709043526678,1.22049830417059,0.7));
#12458=CARTESIAN_POINT('Ctrl Pts',(8.19846709497879,1.19422430779862,0.7));
#12459=CARTESIAN_POINT('Ctrl Pts',(9.09944331332256,1.15544418981837,0.7));
#12460=CARTESIAN_POINT('Ctrl Pts',(10.,1.10900986674273,0.7));
#12461=CARTESIAN_POINT('Ctrl Pts',(7.29793284700474,1.24939875264889,0.7));
#12462=CARTESIAN_POINT('Ctrl Pts',(8.19957769811722,1.22310890030201,0.699999704549177));
#12463=CARTESIAN_POINT('Ctrl Pts',(9.10076698492607,1.18430758604571,0.700000491839571));
#12464=CARTESIAN_POINT('Ctrl Pts',(10.0014871213396,1.13785139984992,0.7));
#12465=CARTESIAN_POINT('Ctrl Pts',(7.29939288958794,1.29948813715084,0.676630595533454));
#12466=CARTESIAN_POINT('Ctrl Pts',(8.20149954052228,1.27317186922949,0.676644146017132));
#12467=CARTESIAN_POINT('Ctrl Pts',(9.10306300621911,1.23433322993607,0.676664155483857));
#12468=CARTESIAN_POINT('Ctrl Pts',(10.0040646682326,1.18784086746588,0.676686753673613));
#12469=CARTESIAN_POINT('Ctrl Pts',(7.29996660609513,1.31917051289423,0.626939603849942));
#12470=CARTESIAN_POINT('Ctrl Pts',(8.20225661204673,1.29285896783792,0.626974637782525));
#12471=CARTESIAN_POINT('Ctrl Pts',(9.10396596140606,1.25402923300358,0.627026849623412));
#12472=CARTESIAN_POINT('Ctrl Pts',(10.0050807923581,1.20754778500352,0.627085325222079));
#12473=CARTESIAN_POINT('Ctrl Pts',(7.29999999953093,1.32031613471704,0.605285370449856));
#12474=CARTESIAN_POINT('Ctrl Pts',(8.20230020786565,1.29401302889245,0.605326714446839));
#12475=CARTESIAN_POINT('Ctrl Pts',(9.10401978846669,1.25519559703033,0.605388684776982));
#12476=CARTESIAN_POINT('Ctrl Pts',(10.0051416645797,1.20872835322339,0.605457722909465));
#12477=CARTESIAN_POINT('',(7.29999999989017,1.22041345054104,0.7));
#12478=CARTESIAN_POINT('Ctrl Pts',(7.29999999978094,1.22041345055303,0.7));
#12479=CARTESIAN_POINT('Ctrl Pts',(7.51641201913776,1.21409884615949,0.7));
#12480=CARTESIAN_POINT('Ctrl Pts',(7.73280095443524,1.20706364503479,0.7));
#12481=CARTESIAN_POINT('Ctrl Pts',(7.94916654146952,1.19937499621344,0.7));
#12482=CARTESIAN_POINT('',(7.29999999953133,1.3203161347307,0.605285370449834));
#12483=CARTESIAN_POINT('Ctrl Pts',(7.29999999989087,1.22041345054982,0.7));
#12484=CARTESIAN_POINT('Ctrl Pts',(7.30000000079355,1.22832360919786,0.699999999740221));
#12485=CARTESIAN_POINT('Ctrl Pts',(7.29999941101664,1.23617007614594,0.699006006469939));
#12486=CARTESIAN_POINT('Ctrl Pts',(7.29999889581476,1.24381267896118,0.697118889344366));
#12487=CARTESIAN_POINT('Ctrl Pts',(7.29999860583198,1.24811433880851,0.696056720321257));
#12488=CARTESIAN_POINT('Ctrl Pts',(7.29999834128398,1.25235147078274,0.694710570513598));
#12489=CARTESIAN_POINT('Ctrl Pts',(7.29999817264931,1.25649739217805,0.693091458416622));
#12490=CARTESIAN_POINT('Ctrl Pts',(7.29999787070862,1.26392067210813,0.690192435210923));
#12491=CARTESIAN_POINT('Ctrl Pts',(7.29999793286912,1.27097116792553,0.686452948287278));
#12492=CARTESIAN_POINT('Ctrl Pts',(7.2999983123982,1.27750284616821,0.681954753865011));
#12493=CARTESIAN_POINT('Ctrl Pts',(7.2999985213788,1.28109939299731,0.679477906983553));
#12494=CARTESIAN_POINT('Ctrl Pts',(7.29999881895966,1.28453837241868,0.676770138671336));
#12495=CARTESIAN_POINT('Ctrl Pts',(7.29999908362886,1.28779148632494,0.673839551409954));
#12496=CARTESIAN_POINT('Ctrl Pts',(7.29999934163235,1.29096267037196,0.670982771155867));
#12497=CARTESIAN_POINT('Ctrl Pts',(7.29999957112158,1.2939379836903,0.667931525418885));
#12498=CARTESIAN_POINT('Ctrl Pts',(7.29999957127586,1.29669488996436,0.664697318929259));
#12499=CARTESIAN_POINT('Ctrl Pts',(7.29999957156178,1.30180432468448,0.658703293276094));
#12500=CARTESIAN_POINT('Ctrl Pts',(7.29999886995656,1.30616650855536,0.652082235935803));
#12501=CARTESIAN_POINT('Ctrl Pts',(7.29999863193158,1.30972187224872,0.644999691185358));
#12502=CARTESIAN_POINT('Ctrl Pts',(7.29999860759325,1.31008541227461,0.644275492840527));
#12503=CARTESIAN_POINT('Ctrl Pts',(7.29999858692673,1.31044047656777,0.643546449710686));
#12504=CARTESIAN_POINT('Ctrl Pts',(7.29999857034625,1.31078697300061,0.642812727646596));
#12505=CARTESIAN_POINT('Ctrl Pts',(7.29999840819729,1.31417553742296,0.635637287305567));
#12506=CARTESIAN_POINT('Ctrl Pts',(7.29999876577208,1.31670951795567,0.628098908385918));
#12507=CARTESIAN_POINT('Ctrl Pts',(7.29999928780719,1.3183355664444,0.620365998324013));
#12508=CARTESIAN_POINT('Ctrl Pts',(7.29999962266353,1.3193785856694,0.615405768714856));
#12509=CARTESIAN_POINT('Ctrl Pts',(7.3,1.32004717656055,0.610364828659741));
#12510=CARTESIAN_POINT('Ctrl Pts',(7.3,1.32031613470337,0.605285370449877));
#12511=CARTESIAN_POINT('',(10.,1.20899340483173,0.605457329065657));
#12512=CARTESIAN_POINT('Ctrl Pts',(9.99999999968202,1.20899340489109,0.605457329065633));
#12513=CARTESIAN_POINT('Ctrl Pts',(9.10058974048747,1.25534320916473,0.605388449123016));
#12514=CARTESIAN_POINT('Ctrl Pts',(8.20058408060299,1.29406305600824,0.605326635812744));
#12515=CARTESIAN_POINT('Ctrl Pts',(7.29999999953093,1.32031613471704,0.605285370449856));
#12516=CARTESIAN_POINT('',(9.99999999523418,1.1090098672342,0.7));
#12517=CARTESIAN_POINT('Ctrl Pts',(9.99999999968202,1.20899340489109,0.605457329065633));
#12518=CARTESIAN_POINT('Ctrl Pts',(9.99999999887489,1.20856043137698,0.613368813757176));
#12519=CARTESIAN_POINT('Ctrl Pts',(9.99999852309337,1.20715974444566,0.621187403383205));
#12520=CARTESIAN_POINT('Ctrl Pts',(9.99999786661901,1.20487567413208,0.628752957409046));
#12521=CARTESIAN_POINT('Ctrl Pts',(9.9999975031266,1.20361097553651,0.63294203403));
#12522=CARTESIAN_POINT('Ctrl Pts',(9.99999733971606,1.20207445367248,0.63705356322819));
#12523=CARTESIAN_POINT('Ctrl Pts',(9.99999742766416,1.20027388348257,0.64105842070465));
#12524=CARTESIAN_POINT('Ctrl Pts',(9.9999975865154,1.19702170610966,0.6482919664668));
#12525=CARTESIAN_POINT('Ctrl Pts',(9.99999868569093,1.19294650045069,0.655099368158521));
#12526=CARTESIAN_POINT('Ctrl Pts',(9.9999991134218,1.18811276085989,0.661317774786376));
#12527=CARTESIAN_POINT('Ctrl Pts',(9.99999919410111,1.18720101282252,0.662490701033652));
#12528=CARTESIAN_POINT('Ctrl Pts',(9.99999924414009,1.18626214680169,0.663642601192937));
#12529=CARTESIAN_POINT('Ctrl Pts',(9.99999924372355,1.18529642131707,0.664772262763739));
#12530=CARTESIAN_POINT('Ctrl Pts',(9.99999924291654,1.18342543943696,0.666960851926287));
#12531=CARTESIAN_POINT('Ctrl Pts',(9.99999905429896,1.18145367213587,0.669066014649603));
#12532=CARTESIAN_POINT('Ctrl Pts',(9.99999879621773,1.17938809187152,0.671084194359814));
#12533=CARTESIAN_POINT('Ctrl Pts',(9.99999808597787,1.17370361260899,0.676638227242868));
#12534=CARTESIAN_POINT('Ctrl Pts',(9.9999969699445,1.16737553754052,0.681473799108647));
#12535=CARTESIAN_POINT('Ctrl Pts',(9.99999660204079,1.16056788011185,0.685537070165577));
#12536=CARTESIAN_POINT('Ctrl Pts',(9.99999636768906,1.15623145667386,0.688125341392612));
#12537=CARTESIAN_POINT('Ctrl Pts',(9.99999638726733,1.15169947441128,0.690399565850749));
#12538=CARTESIAN_POINT('Ctrl Pts',(9.99999666360534,1.14700857532255,0.692336497939236));
#12539=CARTESIAN_POINT('Ctrl Pts',(9.99999709503399,1.13968497812548,0.695360504669253));
#12540=CARTESIAN_POINT('Ctrl Pts',(9.99999815490668,1.13205884654683,0.697530003145419));
#12541=CARTESIAN_POINT('Ctrl Pts',(9.99999900983214,1.12427739544825,0.698775573347137));
#12542=CARTESIAN_POINT('Ctrl Pts',(9.99999956314479,1.11924119569193,0.699581713521624));
#12543=CARTESIAN_POINT('Ctrl Pts',(10.,1.11413933950174,0.7));
#12544=CARTESIAN_POINT('Ctrl Pts',(10.,1.10900986674273,0.7));
#12545=CARTESIAN_POINT('Ctrl Pts',(8.26514054272776,1.18768929227839,0.7));
#12546=CARTESIAN_POINT('Ctrl Pts',(8.84359655063997,1.16547286645366,0.7));
#12547=CARTESIAN_POINT('Ctrl Pts',(9.42188471826001,1.13881853081542,0.7));
#12548=CARTESIAN_POINT('Ctrl Pts',(9.99999999522154,1.10900986698912,0.7));
#12549=CARTESIAN_POINT('Origin',(5.4,-8.11656130105013E-18,0.7));
#12550=CARTESIAN_POINT('',(7.3,-1.22041345053557,0.7));
#12551=CARTESIAN_POINT('Ctrl Pts',(7.94916654049851,-1.19937499624794,0.7));
#12552=CARTESIAN_POINT('Ctrl Pts',(7.73280095382446,-1.20706364505454,0.7));
#12553=CARTESIAN_POINT('Ctrl Pts',(7.51641201888728,-1.21409884616656,0.7));
#12554=CARTESIAN_POINT('Ctrl Pts',(7.29999999989085,-1.22041345054982,0.7));
#12555=CARTESIAN_POINT('',(7.3,-0.712777777777778,0.7));
#12556=CARTESIAN_POINT('',(10.,-1.10900986674244,0.7));
#12557=CARTESIAN_POINT('',(10.,0.653773457742722,0.7));
#12558=CARTESIAN_POINT('Ctrl Pts',(10.,-1.10900986674273,0.7));
#12559=CARTESIAN_POINT('Ctrl Pts',(9.42188472144661,-1.13881853066854,0.7));
#12560=CARTESIAN_POINT('Ctrl Pts',(8.84359655223373,-1.16547286639245,0.7));
#12561=CARTESIAN_POINT('Ctrl Pts',(8.26514054272776,-1.18768929227839,0.7));
#12562=CARTESIAN_POINT('',(7.95,-1.,0.7));
#12563=CARTESIAN_POINT('Origin',(8.1,-1.,0.7));
#12564=CARTESIAN_POINT('',(7.95,1.,0.7));
#12565=CARTESIAN_POINT('Origin',(8.1,1.,0.7));
#12566=CARTESIAN_POINT('',(8.4,-4.89858719658942E-17,0.7));
#12567=CARTESIAN_POINT('Origin',(8.8,0.,0.7));
#12568=CARTESIAN_POINT('Origin',(8.1,-1.,0.8));
#12569=CARTESIAN_POINT('',(7.95,-1.,0.9));
#12570=CARTESIAN_POINT('Origin',(8.1,-1.,0.9));
#12571=CARTESIAN_POINT('',(7.95,-1.,0.8));
#12572=CARTESIAN_POINT('Origin',(2.7,-1.,0.8));
#12573=CARTESIAN_POINT('',(2.55,-1.,0.9));
#12574=CARTESIAN_POINT('Origin',(2.7,-1.,0.9));
#12575=CARTESIAN_POINT('',(2.55,-1.,0.7));
#12576=CARTESIAN_POINT('',(2.55,-1.,0.8));
#12577=CARTESIAN_POINT('Origin',(2.7,-1.,0.7));
#12578=CARTESIAN_POINT('Origin',(2.7,1.,0.8));
#12579=CARTESIAN_POINT('',(2.55,1.,0.9));
#12580=CARTESIAN_POINT('Origin',(2.7,1.,0.9));
#12581=CARTESIAN_POINT('',(2.55,1.,0.7));
#12582=CARTESIAN_POINT('',(2.55,1.,0.8));
#12583=CARTESIAN_POINT('Origin',(2.7,1.,0.7));
#12584=CARTESIAN_POINT('Origin',(8.1,1.,0.8));
#12585=CARTESIAN_POINT('',(7.95,1.,0.9));
#12586=CARTESIAN_POINT('Origin',(8.1,1.,0.9));
#12587=CARTESIAN_POINT('',(7.95,1.,0.8));
#12588=CARTESIAN_POINT('Origin',(2.,0.,0.75));
#12589=CARTESIAN_POINT('',(1.7,3.67394039744206E-17,0.9));
#12590=CARTESIAN_POINT('Origin',(2.,0.,0.9));
#12591=CARTESIAN_POINT('',(1.7,3.67394039744206E-17,0.6));
#12592=CARTESIAN_POINT('',(1.7,3.67394039744206E-17,0.75));
#12593=CARTESIAN_POINT('Origin',(2.,0.,0.6));
#12594=CARTESIAN_POINT('Origin',(2.,0.,0.6));
#12595=CARTESIAN_POINT('',(1.83,-2.0818995585505E-17,0.6));
#12596=CARTESIAN_POINT('Origin',(2.,0.,0.6));
#12597=CARTESIAN_POINT('Origin',(8.8,0.,0.75));
#12598=CARTESIAN_POINT('',(8.5,3.67394039744206E-17,0.9));
#12599=CARTESIAN_POINT('Origin',(8.8,0.,0.9));
#12600=CARTESIAN_POINT('',(8.5,3.67394039744206E-17,0.6));
#12601=CARTESIAN_POINT('',(8.5,3.67394039744206E-17,0.75));
#12602=CARTESIAN_POINT('Origin',(8.8,0.,0.6));
#12603=CARTESIAN_POINT('Origin',(8.8,0.,0.6));
#12604=CARTESIAN_POINT('',(8.63,-2.0818995585505E-17,0.6));
#12605=CARTESIAN_POINT('Origin',(8.8,0.,0.6));
#12606=CARTESIAN_POINT('Origin',(2.,0.,0.45));
#12607=CARTESIAN_POINT('',(1.83,-2.0818995585505E-17,0.32));
#12608=CARTESIAN_POINT('',(1.83,2.0818995585505E-17,0.45));
#12609=CARTESIAN_POINT('Origin',(2.,0.,0.32));
#12610=CARTESIAN_POINT('Origin',(8.8,0.,0.45));
#12611=CARTESIAN_POINT('',(8.63,-2.0818995585505E-17,0.32));
#12612=CARTESIAN_POINT('',(8.63,2.0818995585505E-17,0.45));
#12613=CARTESIAN_POINT('Origin',(8.8,0.,0.32));
#12614=CARTESIAN_POINT('Origin',(10.,-0.62,0.32));
#12615=CARTESIAN_POINT('',(0.200274469199584,-0.62,0.));
#12616=CARTESIAN_POINT('',(0.217044958570157,-0.62,0.32));
#12617=CARTESIAN_POINT('',(0.221783445591644,-0.62,0.410415718550007));
#12618=CARTESIAN_POINT('',(0.,-0.62,0.));
#12619=CARTESIAN_POINT('',(7.7,-0.62,0.));
#12620=CARTESIAN_POINT('',(0.0167704893705732,-0.62,0.32));
#12621=CARTESIAN_POINT('',(0.0220575386407278,-0.62,0.420882909798596));
#12622=CARTESIAN_POINT('',(-0.1,-0.62,0.32));
#12623=CARTESIAN_POINT('Origin',(10.,-0.62,0.32));
#12624=CARTESIAN_POINT('',(0.9,-0.62,0.32));
#12625=CARTESIAN_POINT('',(0.9,-0.62,0.));
#12626=CARTESIAN_POINT('',(0.9,-0.62,0.16));
#12627=CARTESIAN_POINT('',(1.1,-0.62,0.32));
#12628=CARTESIAN_POINT('',(-0.1,-0.62,0.32));
#12629=CARTESIAN_POINT('',(1.1,-0.62,0.));
#12630=CARTESIAN_POINT('',(1.1,-0.62,0.16));
#12631=CARTESIAN_POINT('',(7.7,-0.62,0.));
#12632=CARTESIAN_POINT('Origin',(10.,-0.62,0.32));
#12633=CARTESIAN_POINT('',(3.5,-0.62,0.32));
#12634=CARTESIAN_POINT('',(3.5,-0.62,0.));
#12635=CARTESIAN_POINT('',(3.5,-0.62,0.16));
#12636=CARTESIAN_POINT('',(3.7,-0.62,0.32));
#12637=CARTESIAN_POINT('',(-0.1,-0.62,0.32));
#12638=CARTESIAN_POINT('',(3.7,-0.62,0.));
#12639=CARTESIAN_POINT('',(3.7,-0.62,0.16));
#12640=CARTESIAN_POINT('',(7.7,-0.62,0.));
#12641=CARTESIAN_POINT('Origin',(10.,-0.62,0.32));
#12642=CARTESIAN_POINT('',(7.1,-0.62,0.32));
#12643=CARTESIAN_POINT('',(7.1,-0.62,0.));
#12644=CARTESIAN_POINT('',(7.1,-0.62,0.16));
#12645=CARTESIAN_POINT('',(7.3,-0.62,0.32));
#12646=CARTESIAN_POINT('',(-0.1,-0.62,0.32));
#12647=CARTESIAN_POINT('',(7.3,-0.62,0.));
#12648=CARTESIAN_POINT('',(7.3,-0.62,0.16));
#12649=CARTESIAN_POINT('',(7.7,-0.62,0.));
#12650=CARTESIAN_POINT('Origin',(-0.0999999999999996,0.62,0.32));
#12651=CARTESIAN_POINT('',(0.217044958570158,0.62,0.32));
#12652=CARTESIAN_POINT('',(0.200274469199584,0.62,0.));
#12653=CARTESIAN_POINT('',(0.207951231396534,0.62,0.146481348799182));
#12654=CARTESIAN_POINT('',(0.0167704893705736,0.62,0.32));
#12655=CARTESIAN_POINT('',(10.,0.62,0.32));
#12656=CARTESIAN_POINT('',(0.,0.62,0.));
#12657=CARTESIAN_POINT('',(0.00822532444561912,0.62,0.156948540047771));
#12658=CARTESIAN_POINT('',(2.65,0.62,0.));
#12659=CARTESIAN_POINT('Origin',(-0.0999999999999996,0.62,0.32));
#12660=CARTESIAN_POINT('',(0.9,0.62,0.));
#12661=CARTESIAN_POINT('',(0.9,0.62,0.32));
#12662=CARTESIAN_POINT('',(0.9,0.62,0.16));
#12663=CARTESIAN_POINT('',(1.1,0.62,0.));
#12664=CARTESIAN_POINT('',(2.65,0.62,0.));
#12665=CARTESIAN_POINT('',(1.1,0.62,0.32));
#12666=CARTESIAN_POINT('',(1.1,0.62,0.16));
#12667=CARTESIAN_POINT('',(10.,0.62,0.32));
#12668=CARTESIAN_POINT('Origin',(-0.0999999999999996,0.62,0.32));
#12669=CARTESIAN_POINT('',(3.5,0.62,0.));
#12670=CARTESIAN_POINT('',(3.5,0.62,0.32));
#12671=CARTESIAN_POINT('',(3.5,0.62,0.16));
#12672=CARTESIAN_POINT('',(3.7,0.62,0.));
#12673=CARTESIAN_POINT('',(2.65,0.62,0.));
#12674=CARTESIAN_POINT('',(3.7,0.62,0.32));
#12675=CARTESIAN_POINT('',(3.7,0.62,0.16));
#12676=CARTESIAN_POINT('',(10.,0.62,0.32));
#12677=CARTESIAN_POINT('Origin',(4.95,0.,0.32));
#12678=CARTESIAN_POINT('',(1.6,-4.89858719658941E-17,0.32));
#12679=CARTESIAN_POINT('Origin',(2.,0.,0.32));
#12680=CARTESIAN_POINT('Origin',(4.95,0.,0.32));
#12681=CARTESIAN_POINT('',(8.4,-4.89858719658942E-17,0.32));
#12682=CARTESIAN_POINT('Origin',(8.8,0.,0.32));
#12683=CARTESIAN_POINT('Origin',(4.95,0.,0.32));
#12684=CARTESIAN_POINT('',(0.217044958570157,-0.7,0.32));
#12685=CARTESIAN_POINT('',(0.0167704893705731,-0.7,0.32));
#12686=CARTESIAN_POINT('Origin',(4.95,0.,0.32));
#12687=CARTESIAN_POINT('',(0.9,0.671641708581009,0.32));
#12688=CARTESIAN_POINT('',(1.1,-0.671641708581009,0.32));
#12689=CARTESIAN_POINT('Origin',(4.95,0.,0.32));
#12690=CARTESIAN_POINT('',(3.5,0.723888888888889,0.32));
#12691=CARTESIAN_POINT('',(3.7,-0.723888888888889,0.32));
#12692=CARTESIAN_POINT('Origin',(4.95,0.,0.32));
#12693=CARTESIAN_POINT('',(7.1,0.62,0.32));
#12694=CARTESIAN_POINT('',(7.1,0.712777777777778,0.32));
#12695=CARTESIAN_POINT('',(7.3,0.62,0.32));
#12696=CARTESIAN_POINT('',(10.,0.62,0.32));
#12697=CARTESIAN_POINT('',(7.3,-0.712777777777778,0.32));
#12698=CARTESIAN_POINT('Origin',(-0.0999999999999996,0.62,0.32));
#12699=CARTESIAN_POINT('',(7.1,0.62,0.));
#12700=CARTESIAN_POINT('',(7.1,0.62,0.16));
#12701=CARTESIAN_POINT('',(7.3,0.62,0.));
#12702=CARTESIAN_POINT('',(2.65,0.62,0.));
#12703=CARTESIAN_POINT('',(7.3,0.62,0.16));
#12704=CARTESIAN_POINT('Origin',(10.,1.30754691548544,0.));
#12705=CARTESIAN_POINT('',(10.,1.24211782565704,0.));
#12706=CARTESIAN_POINT('',(10.,-1.24211782565704,0.));
#12707=CARTESIAN_POINT('',(10.,1.30754691548544,0.));
#12708=CARTESIAN_POINT('',(10.,-1.20899340483173,0.605457329065657));
#12709=CARTESIAN_POINT('Ctrl Pts',(10.,-1.20899340483173,0.605457329065657));
#12710=CARTESIAN_POINT('Ctrl Pts',(10.,-1.21451837038612,0.504502771559899));
#12711=CARTESIAN_POINT('Ctrl Pts',(10.,-1.22004249263249,0.403547366186347));
#12712=CARTESIAN_POINT('Ctrl Pts',(10.,-1.23108392958594,0.201728789021226));
#12713=CARTESIAN_POINT('Ctrl Pts',(10.,-1.23660133320922,0.100864020914724));
#12714=CARTESIAN_POINT('Ctrl Pts',(10.,-1.24211782565704,0.));
#12715=CARTESIAN_POINT('Ctrl Pts',(10.,-1.10900986674273,0.7));
#12716=CARTESIAN_POINT('Ctrl Pts',(10.,-1.11692706738765,0.7));
#12717=CARTESIAN_POINT('Ctrl Pts',(9.99999896020971,-1.12478097169818,0.699006158364426));
#12718=CARTESIAN_POINT('Ctrl Pts',(9.99999805494427,-1.13243115645175,0.697118998397561));
#12719=CARTESIAN_POINT('Ctrl Pts',(9.99999754769332,-1.13671781459207,0.696061558623929));
#12720=CARTESIAN_POINT('Ctrl Pts',(9.99999708556116,-1.14094056283945,0.694722610426682));
#12721=CARTESIAN_POINT('Ctrl Pts',(9.99999679002998,-1.14507302265453,0.693112977943955));
#12722=CARTESIAN_POINT('Ctrl Pts',(9.99999625879002,-1.15250143622127,0.690219540062595));
#12723=CARTESIAN_POINT('Ctrl Pts',(9.999996365957,-1.15955821040664,0.686485807665162));
#12724=CARTESIAN_POINT('Ctrl Pts',(9.99999703387985,-1.16609707610076,0.681992895329386));
#12725=CARTESIAN_POINT('Ctrl Pts',(9.99999740034986,-1.16968476316425,0.679527763880215));
#12726=CARTESIAN_POINT('Ctrl Pts',(9.99999792190556,-1.17311627083768,0.676833210412541));
#12727=CARTESIAN_POINT('Ctrl Pts',(9.99999838578331,-1.17636354905877,0.673917165661822));
#12728=CARTESIAN_POINT('Ctrl Pts',(9.99999884023993,-1.17954487655573,0.671060344436104));
#12729=CARTESIAN_POINT('Ctrl Pts',(9.99999924462882,-1.18253006594632,0.668008218820746));
#12730=CARTESIAN_POINT('Ctrl Pts',(9.99999924442301,-1.185296421281,0.664772262763763));
#12731=CARTESIAN_POINT('Ctrl Pts',(9.99999924404215,-1.19041578560695,0.658783864313737));
#12732=CARTESIAN_POINT('Ctrl Pts',(9.99999800949836,-1.19478865237554,0.652167294255586));
#12733=CARTESIAN_POINT('Ctrl Pts',(9.99999759228052,-1.19835462180986,0.645087621913151));
#12734=CARTESIAN_POINT('Ctrl Pts',(9.99999755030119,-1.19871341999785,0.644375284453517));
#12735=CARTESIAN_POINT('Ctrl Pts',(9.9999975145836,-1.19906401030029,0.643658239626438));
#12736=CARTESIAN_POINT('Ctrl Pts',(9.99999748581823,-1.19940630408966,0.642936645100882));
#12737=CARTESIAN_POINT('Ctrl Pts',(9.99999720003888,-1.20280693749908,0.635767720253638));
#12738=CARTESIAN_POINT('Ctrl Pts',(9.9999978299417,-1.20535324884233,0.628234501710241));
#12739=CARTESIAN_POINT('Ctrl Pts',(9.99999874867777,-1.20699142055415,0.62050509267719));
#12740=CARTESIAN_POINT('Ctrl Pts',(9.99999933690345,-1.20804026874419,0.615556297251186));
#12741=CARTESIAN_POINT('Ctrl Pts',(9.99999999916487,-1.20871598809812,0.61052641213707));
#12742=CARTESIAN_POINT('Ctrl Pts',(9.99999999968202,-1.20899340489109,0.605457329065633));
#12743=CARTESIAN_POINT('Ctrl Pts',(10.,1.24211782565704,0.));
#12744=CARTESIAN_POINT('Ctrl Pts',(10.,1.23660053043673,0.100878698875723));
#12745=CARTESIAN_POINT('Ctrl Pts',(10.,1.23108232376984,0.201758145268796));
#12746=CARTESIAN_POINT('Ctrl Pts',(10.,1.22004088630648,0.403576722396156));
#12747=CARTESIAN_POINT('Ctrl Pts',(10.,1.2145175671044,0.504517449470448));
#12748=CARTESIAN_POINT('Ctrl Pts',(10.,1.20899340483173,0.605457329065657));
#12749=CARTESIAN_POINT('Origin',(7.3,-1.42555555555556,0.));
#12750=CARTESIAN_POINT('',(7.3,1.35236351479115,0.));
#12751=CARTESIAN_POINT('',(7.3,-1.42555555555556,0.));
#12752=CARTESIAN_POINT('Ctrl Pts',(7.29999999953133,1.3203161347307,0.605285370449834));
#12753=CARTESIAN_POINT('Ctrl Pts',(7.29999999953133,1.32565322760551,0.504490726585133));
#12754=CARTESIAN_POINT('Ctrl Pts',(7.3,1.33099015509697,0.403695123734478));
#12755=CARTESIAN_POINT('Ctrl Pts',(7.3,1.34167258064689,0.201933969199042));
#12756=CARTESIAN_POINT('Ctrl Pts',(7.3,1.34701817868136,0.100966514951419));
#12757=CARTESIAN_POINT('Ctrl Pts',(7.3,1.35236351479115,0.));
#12758=CARTESIAN_POINT('',(7.29999999953133,-1.3203161347307,0.605285370449834));
#12759=CARTESIAN_POINT('Ctrl Pts',(7.3,-1.32031613470337,0.605285370449877));
#12760=CARTESIAN_POINT('Ctrl Pts',(7.3,-1.31989712778929,0.61319860217968));
#12761=CARTESIAN_POINT('Ctrl Pts',(7.29999916171872,-1.31851071739963,0.621020829077898));
#12762=CARTESIAN_POINT('Ctrl Pts',(7.29999878808195,-1.31624092632926,0.628591660945423));
#12763=CARTESIAN_POINT('Ctrl Pts',(7.29999857947278,-1.31497365483497,0.632818613610392));
#12764=CARTESIAN_POINT('Ctrl Pts',(7.29999848639856,-1.31343001415,0.636967235874856));
#12765=CARTESIAN_POINT('Ctrl Pts',(7.29999853830689,-1.31161789606625,0.641007613679984));
#12766=CARTESIAN_POINT('Ctrl Pts',(7.29999863125487,-1.30837308502546,0.648242386418365));
#12767=CARTESIAN_POINT('Ctrl Pts',(7.29999925734287,-1.30430566789097,0.655052076019481));
#12768=CARTESIAN_POINT('Ctrl Pts',(7.29999949821933,-1.29947941328181,0.661273460789274));
#12769=CARTESIAN_POINT('Ctrl Pts',(7.29999954322,-1.29857776968225,0.662435743389828));
#12770=CARTESIAN_POINT('Ctrl Pts',(7.29999957102613,-1.29764951297213,0.663577423078133));
#12771=CARTESIAN_POINT('Ctrl Pts',(7.2999995707084,-1.29669488998092,0.664697318929248));
#12772=CARTESIAN_POINT('Ctrl Pts',(7.29999957007561,-1.29479368240016,0.666927680549918));
#12773=CARTESIAN_POINT('Ctrl Pts',(7.29999945886743,-1.29278792931167,0.669071688571899));
#12774=CARTESIAN_POINT('Ctrl Pts',(7.29999930790078,-1.2906849717248,0.671125563583336));
#12775=CARTESIAN_POINT('Ctrl Pts',(7.29999889984047,-1.28500071247856,0.676677153447665));
#12776=CARTESIAN_POINT('Ctrl Pts',(7.29999826931494,-1.27867319504519,0.681510485910933));
#12777=CARTESIAN_POINT('Ctrl Pts',(7.29999806345125,-1.27186607945067,0.685571085769401));
#12778=CARTESIAN_POINT('Ctrl Pts',(7.29999793266427,-1.26754145993833,0.688150820039508));
#12779=CARTESIAN_POINT('Ctrl Pts',(7.29999794545359,-1.26302231037287,0.690417984675215));
#12780=CARTESIAN_POINT('Ctrl Pts',(7.29999810371711,-1.25834494218995,0.69234933099425));
#12781=CARTESIAN_POINT('Ctrl Pts',(7.29999835129001,-1.25102809722258,0.695370551698293));
#12782=CARTESIAN_POINT('Ctrl Pts',(7.29999895574222,-1.24340909242398,0.6975375590939));
#12783=CARTESIAN_POINT('Ctrl Pts',(7.29999944081525,-1.2356348173965,0.698780605629559));
#12784=CARTESIAN_POINT('Ctrl Pts',(7.29999975409932,-1.23061380764338,0.699583426311495));
#12785=CARTESIAN_POINT('Ctrl Pts',(7.30000000047446,-1.22552743956586,0.699999999832051));
#12786=CARTESIAN_POINT('Ctrl Pts',(7.29999999989087,-1.22041345054982,0.7));
#12787=CARTESIAN_POINT('',(7.3,-1.35236351479115,0.));
#12788=CARTESIAN_POINT('Ctrl Pts',(7.3,-1.35236351479115,0.));
#12789=CARTESIAN_POINT('Ctrl Pts',(7.3,-1.34701814920095,0.100967071798286));
#12790=CARTESIAN_POINT('Ctrl Pts',(7.3,-1.34167252169398,0.201935082699409));
#12791=CARTESIAN_POINT('Ctrl Pts',(7.3,-1.33099009614589,0.403696237111114));
#12792=CARTESIAN_POINT('Ctrl Pts',(7.29999999953133,-1.32565319812959,0.504491283257837));
#12793=CARTESIAN_POINT('Ctrl Pts',(7.29999999953133,-1.3203161347307,0.605285370449834));
#12794=CARTESIAN_POINT('',(7.3,-1.42555555555556,0.));
#12795=CARTESIAN_POINT('Origin',(3.7,-1.44777777777778,0.));
#12796=CARTESIAN_POINT('',(3.7,1.37924639543935,0.));
#12797=CARTESIAN_POINT('',(3.7,-1.44777777777778,0.));
#12798=CARTESIAN_POINT('',(3.7,1.34735368793805,0.605261457205193));
#12799=CARTESIAN_POINT('Ctrl Pts',(3.7,1.34735368793805,0.605261457205193));
#12800=CARTESIAN_POINT('Ctrl Pts',(3.7,1.35266395147774,0.504488703431434));
#12801=CARTESIAN_POINT('Ctrl Pts',(3.7,1.35797406404029,0.40371594170176));
#12802=CARTESIAN_POINT('Ctrl Pts',(3.7,1.36860496587027,0.201962122597264));
#12803=CARTESIAN_POINT('Ctrl Pts',(3.7,1.37392575452088,0.100981065191366));
#12804=CARTESIAN_POINT('Ctrl Pts',(3.7,1.37924639543935,0.));
#12805=CARTESIAN_POINT('',(3.7,1.24747724070879,0.7));
#12806=CARTESIAN_POINT('Ctrl Pts',(3.7,1.24747724070879,0.7));
#12807=CARTESIAN_POINT('Ctrl Pts',(3.7,1.25538532734776,0.7));
#12808=CARTESIAN_POINT('Ctrl Pts',(3.70000034866643,1.26322972530331,0.699006048248363));
#12809=CARTESIAN_POINT('Ctrl Pts',(3.70000065268588,1.27087026624727,0.697119044026295));
#12810=CARTESIAN_POINT('Ctrl Pts',(3.7000008238479,1.27517186762995,0.696056666371322));
#12811=CARTESIAN_POINT('Ctrl Pts',(3.70000097972585,1.27940891103121,0.694710185093394));
#12812=CARTESIAN_POINT('Ctrl Pts',(3.70000107833511,1.28355469746902,0.693090631030141));
#12813=CARTESIAN_POINT('Ctrl Pts',(3.70000125487464,1.29097687270382,0.690191153635441));
#12814=CARTESIAN_POINT('Ctrl Pts',(3.7000012145424,1.29802606517866,0.686451118058958));
#12815=CARTESIAN_POINT('Ctrl Pts',(3.70000098691147,1.3045562506385,0.681952404110064));
#12816=CARTESIAN_POINT('Ctrl Pts',(3.70000086156653,1.30815209635338,0.679475187900035));
#12817=CARTESIAN_POINT('Ctrl Pts',(3.70000068390876,1.31159030769532,0.676767042898431));
#12818=CARTESIAN_POINT('Ctrl Pts',(3.70000052608992,1.31484259178137,0.673836088143417));
#12819=CARTESIAN_POINT('Ctrl Pts',(3.70000037216713,1.31801458722906,0.670977489418868));
#12820=CARTESIAN_POINT('Ctrl Pts',(3.70000023558528,1.32099045552882,0.667924239810466));
#12821=CARTESIAN_POINT('Ctrl Pts',(3.70000023595245,1.32374763345498,0.664687876924229));
#12822=CARTESIAN_POINT('Ctrl Pts',(3.70000023663259,1.32885491153898,0.658692977181302));
#12823=CARTESIAN_POINT('Ctrl Pts',(3.70000065621025,1.33321474659758,0.652071180203097));
#12824=CARTESIAN_POINT('Ctrl Pts',(3.70000080093706,1.33676785491319,0.644988218508662));
#12825=CARTESIAN_POINT('Ctrl Pts',(3.70000081573428,1.33713113341147,0.644264039153811));
#12826=CARTESIAN_POINT('Ctrl Pts',(3.70000082835625,1.33748593861467,0.643535019157411));
#12827=CARTESIAN_POINT('Ctrl Pts',(3.70000083855542,1.33783217873901,0.642801324492746));
#12828=CARTESIAN_POINT('Ctrl Pts',(3.70000093832019,1.34121897990539,0.63562457699476));
#12829=CARTESIAN_POINT('Ctrl Pts',(3.70000072997693,1.34375116782692,0.628085030530103));
#12830=CARTESIAN_POINT('Ctrl Pts',(3.70000042189378,1.34537558692779,0.6203512574804));
#12831=CARTESIAN_POINT('Ctrl Pts',(3.70000022417294,1.3464181026242,0.615387895628485));
#12832=CARTESIAN_POINT('Ctrl Pts',(3.70000000036652,1.34708586836718,0.6103438638189));
#12833=CARTESIAN_POINT('Ctrl Pts',(3.69999999992214,1.34735368792773,0.6052614572053));
#12834=CARTESIAN_POINT('',(3.7,-1.24747724070944,0.7));
#12835=CARTESIAN_POINT('',(3.7,-0.723888888888889,0.7));
#12836=CARTESIAN_POINT('',(3.7,-1.34735368793805,0.605261457205193));
#12837=CARTESIAN_POINT('Ctrl Pts',(3.69999999992215,-1.34735368792773,0.6052614572053));
#12838=CARTESIAN_POINT('Ctrl Pts',(3.70000000061408,-1.34693666923469,0.613175212866596));
#12839=CARTESIAN_POINT('Ctrl Pts',(3.70000049671034,-1.34555248374866,0.620998392122869));
#12840=CARTESIAN_POINT('Ctrl Pts',(3.70000071566022,-1.34328499565267,0.628570462735333));
#12841=CARTESIAN_POINT('Ctrl Pts',(3.70000083807517,-1.34201724238155,0.632804009674372));
#12842=CARTESIAN_POINT('Ctrl Pts',(3.7000008913247,-1.34047237297042,0.63695909738719));
#12843=CARTESIAN_POINT('Ctrl Pts',(3.70000085837557,-1.33865827982058,0.641005656934072));
#12844=CARTESIAN_POINT('Ctrl Pts',(3.7000007994669,-1.33541492172585,0.648240369034365));
#12845=CARTESIAN_POINT('Ctrl Pts',(3.70000042420685,-1.33134915897915,0.655050234746405));
#12846=CARTESIAN_POINT('Ctrl Pts',(3.70000027984635,-1.32652447879733,0.661271863919233));
#12847=CARTESIAN_POINT('Ctrl Pts',(3.70000025294096,-1.32562527203035,0.662431429080655));
#12848=CARTESIAN_POINT('Ctrl Pts',(3.7000002362737,-1.32469957579387,0.663570491348455));
#12849=CARTESIAN_POINT('Ctrl Pts',(3.70000023630138,-1.32374763346102,0.664687876924223));
#12850=CARTESIAN_POINT('Ctrl Pts',(3.70000023635686,-1.32184039796576,0.666926581264246));
#12851=CARTESIAN_POINT('Ctrl Pts',(3.70000030283857,-1.31982784222224,0.669078323867587));
#12852=CARTESIAN_POINT('Ctrl Pts',(3.70000039320883,-1.31771738411303,0.671139279696989));
#12853=CARTESIAN_POINT('Ctrl Pts',(3.70000063660146,-1.3120333248939,0.676690015307994));
#12854=CARTESIAN_POINT('Ctrl Pts',(3.7000010126336,-1.30570602994251,0.681522474044465));
#12855=CARTESIAN_POINT('Ctrl Pts',(3.70000113724274,-1.29889910811053,0.685582059356066));
#12856=CARTESIAN_POINT('Ctrl Pts',(3.70000121634872,-1.29457784995583,0.688159217808216));
#12857=CARTESIAN_POINT('Ctrl Pts',(3.70000121058612,-1.2900623422215,0.690424215862126));
#12858=CARTESIAN_POINT('Ctrl Pts',(3.70000111831253,-1.28538881676413,0.692353818784707));
#12859=CARTESIAN_POINT('Ctrl Pts',(3.70000097388434,-1.27807373536961,0.695374066040565));
#12860=CARTESIAN_POINT('Ctrl Pts',(3.70000061691996,-1.27045659963863,0.697540160564298));
#12861=CARTESIAN_POINT('Ctrl Pts',(3.7000003304055,-1.26268427129293,0.698782316368755));
#12862=CARTESIAN_POINT('Ctrl Pts',(3.70000014548661,-1.25766794365683,0.699584014420239));
#12863=CARTESIAN_POINT('Ctrl Pts',(3.7,-1.25258637988459,0.7));
#12864=CARTESIAN_POINT('Ctrl Pts',(3.7,-1.24747724070879,0.7));
#12865=CARTESIAN_POINT('',(3.7,-1.37924639543935,0.));
#12866=CARTESIAN_POINT('Ctrl Pts',(3.7,-1.37924639543935,0.));
#12867=CARTESIAN_POINT('Ctrl Pts',(3.7,-1.37392574223662,0.100981298335747));
#12868=CARTESIAN_POINT('Ctrl Pts',(3.7,-1.36860494130098,0.201962588887634));
#12869=CARTESIAN_POINT('Ctrl Pts',(3.7,-1.35797403946962,0.403716407992068));
#12870=CARTESIAN_POINT('Ctrl Pts',(3.7,-1.3526639391921,0.504488936575732));
#12871=CARTESIAN_POINT('Ctrl Pts',(3.7,-1.34735368793805,0.605261457205193));
#12872=CARTESIAN_POINT('',(3.7,-1.44777777777778,0.));
#12873=CARTESIAN_POINT('Origin',(1.1,-1.34328341716202,0.));
#12874=CARTESIAN_POINT('',(1.1,1.27885335043294,0.));
#12875=CARTESIAN_POINT('',(1.1,-1.34328341716202,0.));
#12876=CARTESIAN_POINT('Ctrl Pts',(1.1,1.24553911298206,0.605485603995113));
#12877=CARTESIAN_POINT('Ctrl Pts',(1.1,1.25109559382646,0.504544105903265));
#12878=CARTESIAN_POINT('Ctrl Pts',(1.1,1.25665083308595,0.403601248768354));
#12879=CARTESIAN_POINT('Ctrl Pts',(1.1,1.26775551906787,0.201773573764085));
#12880=CARTESIAN_POINT('Ctrl Pts',(1.1,1.2733051088238,0.100886182270816));
#12881=CARTESIAN_POINT('Ctrl Pts',(1.1,1.27885335043294,0.));
#12882=CARTESIAN_POINT('',(1.1,-1.14549341399195,0.7));
#12883=CARTESIAN_POINT('',(1.1,-0.671641708581009,0.7));
#12884=CARTESIAN_POINT('',(1.1,-1.24553911298206,0.605485603995113));
#12885=CARTESIAN_POINT('Ctrl Pts',(1.09999999916631,-1.24553911263843,0.605485603997431));
#12886=CARTESIAN_POINT('Ctrl Pts',(1.10000000220634,-1.24510362317222,0.61339691285734));
#12887=CARTESIAN_POINT('Ctrl Pts',(1.10000177015643,-1.24370036622144,0.621215229994996));
#12888=CARTESIAN_POINT('Ctrl Pts',(1.10000252895322,-1.24141353486351,0.628780213666851));
#12889=CARTESIAN_POINT('Ctrl Pts',(1.10000294802756,-1.24015054543059,0.632958263090869));
#12890=CARTESIAN_POINT('Ctrl Pts',(1.10000312162076,-1.23861706177488,0.637059070655947));
#12891=CARTESIAN_POINT('Ctrl Pts',(1.10000299297862,-1.23682078380192,0.641053713130525));
#12892=CARTESIAN_POINT('Ctrl Pts',(1.10000275999609,-1.23356756237267,0.64828837095969));
#12893=CARTESIAN_POINT('Ctrl Pts',(1.10000138715103,-1.22949085733774,0.655096441442141));
#12894=CARTESIAN_POINT('Ctrl Pts',(1.10000084482056,-1.2246552743941,0.661315040399663));
#12895=CARTESIAN_POINT('Ctrl Pts',(1.10000074196669,-1.22373819809959,0.662494407966206));
#12896=CARTESIAN_POINT('Ctrl Pts',(1.1000006773267,-1.22279369438101,0.663652502541609));
#12897=CARTESIAN_POINT('Ctrl Pts',(1.10000067553493,-1.22182202641035,0.66478809188211));
#12898=CARTESIAN_POINT('Ctrl Pts',(1.10000067210542,-1.219962222636,0.666961646435043));
#12899=CARTESIAN_POINT('Ctrl Pts',(1.10000089707048,-1.21800293160495,0.669052796220007));
#12900=CARTESIAN_POINT('Ctrl Pts',(1.10000120920309,-1.21595100691259,0.671058078730413));
#12901=CARTESIAN_POINT('Ctrl Pts',(1.10000207391986,-1.21026645613745,0.676613414309409));
#12902=CARTESIAN_POINT('Ctrl Pts',(1.1000034579227,-1.20393786500476,0.681450029097565));
#12903=CARTESIAN_POINT('Ctrl Pts',(1.10000394126019,-1.19712964857754,0.685514663758263));
#12904=CARTESIAN_POINT('Ctrl Pts',(1.10000424974863,-1.19278432848208,0.688108902478585));
#12905=CARTESIAN_POINT('Ctrl Pts',(1.10000425197701,-1.18824265871575,0.690387991283085));
#12906=CARTESIAN_POINT('Ctrl Pts',(1.10000394032285,-1.18354156621637,0.692328715646671));
#12907=CARTESIAN_POINT('Ctrl Pts',(1.10000345443802,-1.17621232165581,0.695354404566264));
#12908=CARTESIAN_POINT('Ctrl Pts',(1.10000219938511,-1.16858027633095,0.697525330589554));
#12909=CARTESIAN_POINT('Ctrl Pts',(1.10000118192936,-1.16079305972554,0.698772417158578));
#12910=CARTESIAN_POINT('Ctrl Pts',(1.10000052251962,-1.15574619011492,0.699580649884844));
#12911=CARTESIAN_POINT('Ctrl Pts',(1.1,-1.15063354328712,0.7));
#12912=CARTESIAN_POINT('Ctrl Pts',(1.1,-1.14549341399196,0.7));
#12913=CARTESIAN_POINT('',(1.1,-1.27885335043294,0.));
#12914=CARTESIAN_POINT('Ctrl Pts',(1.1,-1.27885335043294,0.));
#12915=CARTESIAN_POINT('Ctrl Pts',(1.1,-1.27330503870861,0.100887457206881));
#12916=CARTESIAN_POINT('Ctrl Pts',(1.1,-1.26775537880223,0.201776123688554));
#12917=CARTESIAN_POINT('Ctrl Pts',(1.1,-1.25665069275548,0.403603798678134));
#12918=CARTESIAN_POINT('Ctrl Pts',(1.1,-1.25109552364596,0.504545380833391));
#12919=CARTESIAN_POINT('Ctrl Pts',(1.1,-1.24553911298206,0.605485603995113));
#12920=CARTESIAN_POINT('',(1.1,-1.34328341716202,0.));
#12921=CARTESIAN_POINT('Origin',(0.199725906950915,-1.4,-0.0104671912485888));
#12922=CARTESIAN_POINT('',(0.200274469199584,1.12301388185427,1.38777878078145E-17));
#12923=CARTESIAN_POINT('',(0.200274469199585,-0.7,0.));
#12924=CARTESIAN_POINT('',(0.231993417893744,1.09142177001972,0.605233595624295));
#12925=CARTESIAN_POINT('Ctrl Pts',(0.200274469199584,1.12301388185427,-2.97071395261028E-17));
#12926=CARTESIAN_POINT('Ctrl Pts',(0.210847451470635,1.11248294808,0.201744519910852));
#12927=CARTESIAN_POINT('Ctrl Pts',(0.22142043436526,1.101952242875,0.403489051720196));
#12928=CARTESIAN_POINT('Ctrl Pts',(0.231993417893744,1.09142177001972,0.605233595624295));
#12929=CARTESIAN_POINT('',(0.231993417893744,-1.09142177001972,0.605233595624295));
#12930=CARTESIAN_POINT('',(0.231993417893744,-0.7,0.605233595624295));
#12931=CARTESIAN_POINT('',(0.200274469199584,-1.12301388185427,-1.38777878078145E-17));
#12932=CARTESIAN_POINT('Ctrl Pts',(0.231993417893744,-1.09142177001972,
0.605233595624295));
#12933=CARTESIAN_POINT('Ctrl Pts',(0.22142043436526,-1.101952242875,0.403489051720196));
#12934=CARTESIAN_POINT('Ctrl Pts',(0.210847451470635,-1.11248294808,0.201744519910852));
#12935=CARTESIAN_POINT('Ctrl Pts',(0.200274469199584,-1.12301388185427,
-4.90059381963448E-17));
#12936=CARTESIAN_POINT('',(0.200274469199585,-0.7,0.));
#12937=CARTESIAN_POINT('Origin',(5.4,-1.11022302462516E-16,0.));
#12938=CARTESIAN_POINT('Ctrl Pts',(7.29999999999999,-1.35236351479115,1.04083408558608E-17));
#12939=CARTESIAN_POINT('Ctrl Pts',(8.20044803681595,-1.32637404707459,3.18306896032855E-8));
#12940=CARTESIAN_POINT('Ctrl Pts',(9.10060048441536,-1.28803709316692,1.03188250195688E-8));
#12941=CARTESIAN_POINT('Ctrl Pts',(10.0000000000405,-1.24211782537639,-8.23328475353175E-12));
#12942=CARTESIAN_POINT('Ctrl Pts',(10.0000000000405,1.24211782537639,-8.23320567538283E-12));
#12943=CARTESIAN_POINT('Ctrl Pts',(9.1006004808701,1.28803709334794,1.03184817085883E-8));
#12944=CARTESIAN_POINT('Ctrl Pts',(8.20044803144508,1.32637404722969,3.18291413954212E-8));
#12945=CARTESIAN_POINT('Ctrl Pts',(7.3,1.35236351479115,4.75121773919879E-17));
#12946=CARTESIAN_POINT('',(7.1,1.35793097395724,0.));
#12947=CARTESIAN_POINT('',(7.1,1.42555555555556,0.));
#12948=CARTESIAN_POINT('Ctrl Pts',(7.1000000000396,1.35793097389613,-4.88924676637329E-12));
#12949=CARTESIAN_POINT('Ctrl Pts',(6.53177385320612,1.37316067096195,3.71763852401782E-9));
#12950=CARTESIAN_POINT('Ctrl Pts',(5.96344379069665,1.38333257666104,-3.82408184804385E-8));
#12951=CARTESIAN_POINT('Ctrl Pts',(5.39512359652123,1.38725406840392,-3.97623797275691E-8));
#12952=CARTESIAN_POINT('Ctrl Pts',(4.82973248928002,1.39115534902226,-4.12760989429076E-8));
#12953=CARTESIAN_POINT('Ctrl Pts',(4.26470859812609,1.38886839226708,1.63957607983357E-8));
#12954=CARTESIAN_POINT('Ctrl Pts',(3.70000000036239,1.37924639538501,-6.25376529969227E-12));
#12955=CARTESIAN_POINT('',(3.5,1.37552980833516,0.));
#12956=CARTESIAN_POINT('',(3.5,1.44777777777778,0.));
#12957=CARTESIAN_POINT('Ctrl Pts',(3.50000000097466,1.37552980835479,1.06251812903579E-15));
#12958=CARTESIAN_POINT('Ctrl Pts',(2.69943075695685,1.35940904975719,2.35366119539541E-7));
#12959=CARTESIAN_POINT('Ctrl Pts',(1.89948254587541,1.32827224396921,2.51300192353997E-7));
#12960=CARTESIAN_POINT('Ctrl Pts',(1.10000000028363,1.27885335028943,-5.13283415455519E-11));
#12961=CARTESIAN_POINT('',(0.9,1.266106713614,0.));
#12962=CARTESIAN_POINT('',(0.9,1.34328341716202,0.));
#12963=CARTESIAN_POINT('',(0.292382661757373,1.22257596919059,0.));
#12964=CARTESIAN_POINT('Ctrl Pts',(0.9,1.266106713614,1.20346441145891E-16));
#12965=CARTESIAN_POINT('Ctrl Pts',(0.697432754539207,1.25280566772398,-2.10387859372414E-8));
#12966=CARTESIAN_POINT('Ctrl Pts',(0.494894520889663,1.23831317328004,3.6654767345328E-12));
#12967=CARTESIAN_POINT('Ctrl Pts',(0.292382661757371,1.22257596919059,2.98331735103528E-16));
#12968=CARTESIAN_POINT('Ctrl Pts',(0.292382661757373,1.22257596919059,2.94902990916057E-17));
#12969=CARTESIAN_POINT('Ctrl Pts',(0.284469747869226,1.22196105627757,-8.65621238729993E-13));
#12970=CARTESIAN_POINT('Ctrl Pts',(0.276673396002317,1.22038240716686,-1.19564355630166E-6));
#12971=CARTESIAN_POINT('Ctrl Pts',(0.269153172408756,1.21792571627104,-1.29137975931779E-6));
#12972=CARTESIAN_POINT('Ctrl Pts',(0.264330998492885,1.21635041859408,-1.35276844214688E-6));
#12973=CARTESIAN_POINT('Ctrl Pts',(0.259622238853914,1.21441292414196,-1.0165784587106E-6));
#12974=CARTESIAN_POINT('Ctrl Pts',(0.255072584042237,1.21212521597766,-4.21167369976509E-7));
#12975=CARTESIAN_POINT('Ctrl Pts',(0.247984787860257,1.20856125126747,5.06409032217246E-7));
#12976=CARTESIAN_POINT('Ctrl Pts',(0.241364979299678,1.20419126978451,2.25366520907849E-6));
#12977=CARTESIAN_POINT('Ctrl Pts',(0.235375785094684,1.19908071490398,1.28723124315333E-6));
#12978=CARTESIAN_POINT('Ctrl Pts',(0.235058634311792,1.19881009144014,1.23605486142058E-6));
#12979=CARTESIAN_POINT('Ctrl Pts',(0.234743258170683,1.19853738091759,1.17639378419006E-6));
#12980=CARTESIAN_POINT('Ctrl Pts',(0.234429683218046,1.19826258967301,1.10742116603597E-6));
#12981=CARTESIAN_POINT('Ctrl Pts',(0.23095881299434,1.19522100506769,3.4398325561458E-7));
#12982=CARTESIAN_POINT('Ctrl Pts',(0.227708211416394,1.19192479473749,-1.52348441667556E-6));
#12983=CARTESIAN_POINT('Ctrl Pts',(0.224692430858345,1.18840300965977,-3.42436181452249E-6));
#12984=CARTESIAN_POINT('Ctrl Pts',(0.219522873151367,1.18236607466387,-6.68278702580898E-6));
#12985=CARTESIAN_POINT('Ctrl Pts',(0.21509942609515,1.17573654654733,-9.78259773483875E-6));
#12986=CARTESIAN_POINT('Ctrl Pts',(0.211478909386775,1.16867548752938,-1.04320859863301E-5));
#12987=CARTESIAN_POINT('Ctrl Pts',(0.20968494559888,1.16517673715679,-1.075390701291E-5));
#12988=CARTESIAN_POINT('Ctrl Pts',(0.208088728862602,1.16157146972622,-1.05358292927083E-5));
#12989=CARTESIAN_POINT('Ctrl Pts',(0.206701335101202,1.15787708229469,-9.83193564179307E-6));
#12990=CARTESIAN_POINT('Ctrl Pts',(0.203919119965097,1.15046852899383,-8.42037994342582E-6));
#12991=CARTESIAN_POINT('Ctrl Pts',(0.202003457218558,1.1427818296106,-4.88542801801716E-6));
#12992=CARTESIAN_POINT('Ctrl Pts',(0.201024541128784,1.13496408391561,-2.30807221316776E-6));
#12993=CARTESIAN_POINT('Ctrl Pts',(0.200529226009753,1.13100843574523,-1.00397341389412E-6));
#12994=CARTESIAN_POINT('Ctrl Pts',(0.200274469344113,1.12701892049093,-1.14168925800036E-11));
#12995=CARTESIAN_POINT('Ctrl Pts',(0.200274469199584,1.12301388185427,-1.43114686768087E-17));
#12996=CARTESIAN_POINT('',(-1.73234772679968E-18,1.12356026268968,4.53319947845445E-20));
#12997=CARTESIAN_POINT('',(0.,-1.4,0.));
#12998=CARTESIAN_POINT('',(0.276326924564679,1.42224670711126,-2.77555756156289E-17));
#12999=CARTESIAN_POINT('Ctrl Pts',(0.276326924564681,1.42224670711126,-1.50920942409982E-16));
#13000=CARTESIAN_POINT('Ctrl Pts',(0.258529852003869,1.4208638358667,-3.32972379743633E-13));
#13001=CARTESIAN_POINT('Ctrl Pts',(0.240927013527826,1.41785398988725,-1.99727536601662E-6));
#13002=CARTESIAN_POINT('Ctrl Pts',(0.223720619657732,1.41333325652174,-2.71091968639774E-6));
#13003=CARTESIAN_POINT('Ctrl Pts',(0.206313289378911,1.40875972999491,-3.432897951005E-6));
#13004=CARTESIAN_POINT('Ctrl Pts',(0.18931019325249,1.40263932318529,-2.78724979559428E-6));
#13005=CARTESIAN_POINT('Ctrl Pts',(0.172932985028856,1.39504220432096,-6.31841720307455E-7));
#13006=CARTESIAN_POINT('Ctrl Pts',(0.170060146426803,1.39370954151055,-2.53746782677961E-7));
#13007=CARTESIAN_POINT('Ctrl Pts',(0.167206630967902,1.39233132643846,1.61597591574489E-7));
#13008=CARTESIAN_POINT('Ctrl Pts',(0.164373729059928,1.39090779908693,6.02790108062464E-7));
#13009=CARTESIAN_POINT('Ctrl Pts',(0.148213121449433,1.38278712717586,3.11962244863226E-6));
#13010=CARTESIAN_POINT('Ctrl Pts',(0.132864864406694,1.37326763401578,6.8005293729143E-6));
#13011=CARTESIAN_POINT('Ctrl Pts',(0.118540368157823,1.36244192017091,7.47011412280372E-6));
#13012=CARTESIAN_POINT('Ctrl Pts',(0.1130124780146,1.35826422653222,7.72851001154276E-6));
#13013=CARTESIAN_POINT('Ctrl Pts',(0.107637267132642,1.35389150739715,7.50091387420595E-6));
#13014=CARTESIAN_POINT('Ctrl Pts',(0.102427993107927,1.34932731552598,6.39696583889361E-6));
#13015=CARTESIAN_POINT('Ctrl Pts',(0.0920147884934566,1.34020361352282,
4.19020214765608E-6));
#13016=CARTESIAN_POINT('Ctrl Pts',(0.082263696775192,1.33031540618347,-1.43705507633734E-6));
#13017=CARTESIAN_POINT('Ctrl Pts',(0.0732179607829324,1.31975004019149,
-7.24116446069057E-6));
#13018=CARTESIAN_POINT('Ctrl Pts',(0.0614369648181435,1.30598990677343,
-1.48003270644599E-5));
#13019=CARTESIAN_POINT('Ctrl Pts',(0.0509520748529884,1.29120077200215,
-2.24515165560165E-5));
#13020=CARTESIAN_POINT('Ctrl Pts',(0.0418305631051555,1.27560026299671,
-2.64881615939377E-5));
#13021=CARTESIAN_POINT('Ctrl Pts',(0.0329966685655992,1.26049166530727,
-3.03975241584371E-5));
#13022=CARTESIAN_POINT('Ctrl Pts',(0.0254411283904758,1.24462062939249,
-3.09701348507133E-5));
#13023=CARTESIAN_POINT('Ctrl Pts',(0.0192647836588538,1.2281607987719,-2.81763116144976E-5));
#13024=CARTESIAN_POINT('Ctrl Pts',(0.0129258683931997,1.2112677210496,-2.53089508159798E-5));
#13025=CARTESIAN_POINT('Ctrl Pts',(0.00809110271874438,1.19389182855556,
-1.89493195503086E-5));
#13026=CARTESIAN_POINT('Ctrl Pts',(0.00484442764459327,1.17622983835018,
-1.25518552566888E-5));
#13027=CARTESIAN_POINT('Ctrl Pts',(0.00165723550742335,1.1588914367474,
-6.27160009448058E-6));
#13028=CARTESIAN_POINT('Ctrl Pts',(1.90718451428807E-9,1.14127598190669,
-1.51296892603399E-10));
#13029=CARTESIAN_POINT('Ctrl Pts',(2.41777084464267E-17,1.12356026268968,
-3.46944695195361E-18));
#13030=CARTESIAN_POINT('',(10.5166159648474,1.4155315881283,0.));
#13031=CARTESIAN_POINT('Ctrl Pts',(0.276326924564679,1.42224670711126,0.));
#13032=CARTESIAN_POINT('Ctrl Pts',(3.68975660465893,1.68747752195839,0.));
#13033=CARTESIAN_POINT('Ctrl Pts',(7.10318628475318,1.599994843061,0.));
#13034=CARTESIAN_POINT('Ctrl Pts',(10.5166159648474,1.4155315881283,0.));
#13035=CARTESIAN_POINT('',(10.8,1.11638029377732,-5.56631991785941E-17));
#13036=CARTESIAN_POINT('Ctrl Pts',(10.8,1.11638029377732,2.32452945780892E-16));
#13037=CARTESIAN_POINT('Ctrl Pts',(10.7999999994302,1.13421844616111,-9.29296349749781E-12));
#13038=CARTESIAN_POINT('Ctrl Pts',(10.7983603663884,1.15198349698667,-2.38856955364628E-6));
#13039=CARTESIAN_POINT('Ctrl Pts',(10.7951843826221,1.16946861094468,-3.77014304120448E-6));
#13040=CARTESIAN_POINT('Ctrl Pts',(10.7919669771209,1.18718176881198,-5.16973525142236E-6));
#13041=CARTESIAN_POINT('Ctrl Pts',(10.7871724978816,1.20460918321158,-5.4755482503851E-6));
#13042=CARTESIAN_POINT('Ctrl Pts',(10.7808573412527,1.22152732075962,-4.27334038376583E-6));
#13043=CARTESIAN_POINT('Ctrl Pts',(10.7797421066656,1.22451500471617,-4.06103467663179E-6));
#13044=CARTESIAN_POINT('Ctrl Pts',(10.7785793293545,1.22748675045939,-3.81081650224554E-6));
#13045=CARTESIAN_POINT('Ctrl Pts',(10.7773691713543,1.23044124224994,-3.53261416912234E-6));
#13046=CARTESIAN_POINT('Ctrl Pts',(10.7705159051166,1.24717287467681,-1.95712183132163E-6));
#13047=CARTESIAN_POINT('Ctrl Pts',(10.7622076549587,1.26320448426569,8.50150473021234E-7));
#13048=CARTESIAN_POINT('Ctrl Pts',(10.7525236566209,1.27832128496499,1.09915986206012E-6));
#13049=CARTESIAN_POINT('Ctrl Pts',(10.7482509716548,1.28499098118248,1.20902550183604E-6));
#13050=CARTESIAN_POINT('Ctrl Pts',(10.7437098328292,1.29148238441373,7.76315258636623E-7));
#13051=CARTESIAN_POINT('Ctrl Pts',(10.7389041877712,1.29777551763099,-7.54184826032082E-7));
#13052=CARTESIAN_POINT('Ctrl Pts',(10.7310976851069,1.30799836193882,-3.24039694621926E-6));
#13053=CARTESIAN_POINT('Ctrl Pts',(10.7225935645301,1.31769858917671,-8.57388820182801E-6));
#13054=CARTESIAN_POINT('Ctrl Pts',(10.7134588931078,1.3268364513864,-1.41086939541967E-5));
#13055=CARTESIAN_POINT('Ctrl Pts',(10.7004433550849,1.33985653580309,-2.19949628070403E-5));
#13056=CARTESIAN_POINT('Ctrl Pts',(10.6862650266646,1.35162127070648,-3.0022236679635E-5));
#13057=CARTESIAN_POINT('Ctrl Pts',(10.6711476119081,1.36204513612776,-3.40981369893719E-5));
#13058=CARTESIAN_POINT('Ctrl Pts',(10.6560301971515,1.37246900154903,-3.81740372991087E-5));
#13059=CARTESIAN_POINT('Ctrl Pts',(10.6399721826852,1.38155285075117,-3.83332859284948E-5));
#13060=CARTESIAN_POINT('Ctrl Pts',(10.6231652498763,1.38916602817047,-3.45204725343976E-5));
#13061=CARTESIAN_POINT('Ctrl Pts',(10.6063487480974,1.39678354012646,-3.07054883279539E-5));
#13062=CARTESIAN_POINT('Ctrl Pts',(10.5889271210941,1.40286310406803,-2.29928881382306E-5));
#13063=CARTESIAN_POINT('Ctrl Pts',(10.5711041279812,1.40730078588308,-1.53078138731408E-5));
#13064=CARTESIAN_POINT('Ctrl Pts',(10.5532811348684,1.41173846769814,-7.6227396080509E-6));
#13065=CARTESIAN_POINT('Ctrl Pts',(10.5350552605908,1.41453511891929,-9.16729947674095E-11));
#13066=CARTESIAN_POINT('Ctrl Pts',(10.5166159648474,1.4155315881283,2.48932818802672E-16));
#13067=CARTESIAN_POINT('',(10.8,-1.11638029377732,-1.39157997946485E-17));
#13068=CARTESIAN_POINT('',(10.8,1.4,0.));
#13069=CARTESIAN_POINT('',(10.5166159648474,-1.4155315881283,2.77555756156289E-17));
#13070=CARTESIAN_POINT('Ctrl Pts',(10.5166159648474,-1.4155315881283,-1.94289029309402E-16));
#13071=CARTESIAN_POINT('Ctrl Pts',(10.5344251606169,-1.41456917089032,1.72780596414851E-12));
#13072=CARTESIAN_POINT('Ctrl Pts',(10.5520727686739,-1.41197333457428,-2.53403886306205E-6));
#13073=CARTESIAN_POINT('Ctrl Pts',(10.5693578805681,-1.40785843881911,-4.04156906196095E-6));
#13074=CARTESIAN_POINT('Ctrl Pts',(10.5868701251756,-1.40368947182374,-5.56890876087065E-6));
#13075=CARTESIAN_POINT('Ctrl Pts',(10.604011804524,-1.39796079212135,-5.98742339745246E-6));
#13076=CARTESIAN_POINT('Ctrl Pts',(10.6205627760847,-1.39074087128671,-4.81856832951796E-6));
#13077=CARTESIAN_POINT('Ctrl Pts',(10.6234754753687,-1.38947028374636,-4.61286902618664E-6));
#13078=CARTESIAN_POINT('Ctrl Pts',(10.6263698187278,-1.38815339768352,-4.36721670635639E-6));
#13079=CARTESIAN_POINT('Ctrl Pts',(10.629244514885,-1.38679044403738,-4.09122931699412E-6));
#13080=CARTESIAN_POINT('Ctrl Pts',(10.6455827855986,-1.37904412775797,-2.5226612199239E-6));
#13081=CARTESIAN_POINT('Ctrl Pts',(10.6611432679573,-1.36988219838444,3.58605122725343E-7));
#13082=CARTESIAN_POINT('Ctrl Pts',(10.6757157985124,-1.35939560704671,7.40589063327193E-7));
#13083=CARTESIAN_POINT('Ctrl Pts',(10.6821516119741,-1.35476430808026,9.09288478831296E-7));
#13084=CARTESIAN_POINT('Ctrl Pts',(10.6883944859408,-1.34987400891586,5.44816430868337E-7));
#13085=CARTESIAN_POINT('Ctrl Pts',(10.6944246343503,-1.34472976213865,-9.14752338109426E-7));
#13086=CARTESIAN_POINT('Ctrl Pts',(10.7041966733629,-1.33639335368171,-3.28002794718031E-6));
#13087=CARTESIAN_POINT('Ctrl Pts',(10.7134106653983,-1.3273903805878,-8.47259327327479E-6));
#13088=CARTESIAN_POINT('Ctrl Pts',(10.7220307555455,-1.31778973409553,-1.38734771921913E-5));
#13089=CARTESIAN_POINT('Ctrl Pts',(10.7343338492722,-1.3040871333553,-2.15819326638919E-5));
#13090=CARTESIAN_POINT('Ctrl Pts',(10.7453199276401,-1.28929041974124,-2.94555326738194E-5));
#13091=CARTESIAN_POINT('Ctrl Pts',(10.7549158277293,-1.27362793268665,-3.3443536645081E-5));
#13092=CARTESIAN_POINT('Ctrl Pts',(10.7645117278185,-1.25796544563206,-3.74315406163426E-5));
#13093=CARTESIAN_POINT('Ctrl Pts',(10.7727182208071,-1.24143562566754,-3.75750290962259E-5));
#13094=CARTESIAN_POINT('Ctrl Pts',(10.7794153247677,-1.22423716044977,-3.38265125308188E-5));
#13095=CARTESIAN_POINT('Ctrl Pts',(10.7861166764432,-1.20702778690835,-3.00756184258222E-5));
#13096=CARTESIAN_POINT('Ctrl Pts',(10.7912490477072,-1.18929683429644,-2.25107044755726E-5));
#13097=CARTESIAN_POINT('Ctrl Pts',(10.7947196858669,-1.17125359626911,-1.49815203503087E-5));
#13098=CARTESIAN_POINT('Ctrl Pts',(10.7981903240266,-1.15321035824179,-7.45233622504479E-6));
#13099=CARTESIAN_POINT('Ctrl Pts',(10.7999999985278,-1.13485327409571,-1.17780195603766E-10));
#13100=CARTESIAN_POINT('Ctrl Pts',(10.8,-1.11638029377732,-1.38777878078145E-17));
#13101=CARTESIAN_POINT('',(0.276326924564679,-1.42224670711126,-5.55111512312578E-17));
#13102=CARTESIAN_POINT('Ctrl Pts',(10.5166159648474,-1.4155315881283,0.));
#13103=CARTESIAN_POINT('Ctrl Pts',(7.10318628475318,-1.599994843061,0.));
#13104=CARTESIAN_POINT('Ctrl Pts',(3.68975660465893,-1.68747752195839,0.));
#13105=CARTESIAN_POINT('Ctrl Pts',(0.276326924564679,-1.42224670711126,
0.));
#13106=CARTESIAN_POINT('',(-7.25311916552711E-19,-1.12356026268968,1.39157997946485E-17));
#13107=CARTESIAN_POINT('Ctrl Pts',(1.80411241501588E-16,-1.12356026268968,
-1.53523027623947E-16));
#13108=CARTESIAN_POINT('Ctrl Pts',(7.41078168374529E-10,-1.14141522098415,
-1.3067981184062E-11));
#13109=CARTESIAN_POINT('Ctrl Pts',(0.00163694718329378,-1.15920272117896,
-1.78823819589733E-6));
#13110=CARTESIAN_POINT('Ctrl Pts',(0.00481087395297265,-1.17671209893291,
-2.3181425555783E-6));
#13111=CARTESIAN_POINT('Ctrl Pts',(0.00802138847203439,-1.19442331774104,
-2.85415543927884E-6));
#13112=CARTESIAN_POINT('Ctrl Pts',(0.0128049030182357,-1.21185152247087,
-2.04128886843626E-6));
#13113=CARTESIAN_POINT('Ctrl Pts',(0.0191087770915565,-1.22877027194193,
1.71240493184593E-7));
#13114=CARTESIAN_POINT('Ctrl Pts',(0.0202201941454154,-1.23175316571065,
5.613248819379E-7));
#13115=CARTESIAN_POINT('Ctrl Pts',(0.0213789882593307,-1.23472016785247,
9.85829603970989E-7));
#13116=CARTESIAN_POINT('Ctrl Pts',(0.0225850188675993,-1.23766995297306,
1.43287414332239E-6));
#13117=CARTESIAN_POINT('Ctrl Pts',(0.0294291562303479,-1.25440977235863,
3.96981990042924E-6));
#13118=CARTESIAN_POINT('Ctrl Pts',(0.0377300686697735,-1.27044838970616,
7.55798501181421E-6));
#13119=CARTESIAN_POINT('Ctrl Pts',(0.0474121614036163,-1.28556782977674,
8.05058320302158E-6));
#13120=CARTESIAN_POINT('Ctrl Pts',(0.0511425121829324,-1.29139310088294,
8.24037316857697E-6));
#13121=CARTESIAN_POINT('Ctrl Pts',(0.0550784035723718,-1.29708174651376,
7.93435480917585E-6));
#13122=CARTESIAN_POINT('Ctrl Pts',(0.0592173503759339,-1.30262033374061,
6.74858081742264E-6));
#13123=CARTESIAN_POINT('Ctrl Pts',(0.0675201807396794,-1.31373087764993,
4.36988865960166E-6));
#13124=CARTESIAN_POINT('Ctrl Pts',(0.0766394565597649,-1.32423847988766,
-1.46587651676554E-6));
#13125=CARTESIAN_POINT('Ctrl Pts',(0.0864911062490747,-1.33409287340636,
-7.46705500292641E-6));
#13126=CARTESIAN_POINT('Ctrl Pts',(0.0992988409846585,-1.34690417528452,
-1.52689465211603E-5));
#13127=CARTESIAN_POINT('Ctrl Pts',(0.113232871116931,-1.35850278376499,
-2.31308069859054E-5));
#13128=CARTESIAN_POINT('Ctrl Pts',(0.128081622025101,-1.36880445085772,
-2.72849174168177E-5));
#13129=CARTESIAN_POINT('Ctrl Pts',(0.142447925282442,-1.37877140864598,
-3.13040575171566E-5));
#13130=CARTESIAN_POINT('Ctrl Pts',(0.157671864768995,-1.38752483454192,
-3.1899138628041E-5));
#13131=CARTESIAN_POINT('Ctrl Pts',(0.173588691395025,-1.39495074934422,
-2.90326641197332E-5));
#13132=CARTESIAN_POINT('Ctrl Pts',(0.189936400238013,-1.40257769006131,
-2.60885916756054E-5));
#13133=CARTESIAN_POINT('Ctrl Pts',(0.206881864105471,-1.40874232120582,
-1.95409011442111E-5));
#13134=CARTESIAN_POINT('Ctrl Pts',(0.22423558959196,-1.41334558507228,-1.29462590315495E-5));
#13135=CARTESIAN_POINT('Ctrl Pts',(0.241260467995769,-1.4178616186841,-6.47658310103417E-6));
#13136=CARTESIAN_POINT('Ctrl Pts',(0.258679581942429,-1.42087546890512,
-1.12101563992788E-10));
#13137=CARTESIAN_POINT('Ctrl Pts',(0.27632692456468,-1.42224670711126,1.05818132034585E-16));
#13138=CARTESIAN_POINT('',(0.,-1.4,0.));
#13139=CARTESIAN_POINT('',(0.292382661757373,-1.22257596919059,0.));
#13140=CARTESIAN_POINT('Ctrl Pts',(0.200274469199584,-1.12301388185427,
-2.68882138776405E-17));
#13141=CARTESIAN_POINT('Ctrl Pts',(0.200274469314753,-1.13095194822878,
-2.85686379674833E-12));
#13142=CARTESIAN_POINT('Ctrl Pts',(0.201244085522878,-1.13884856843413,
-1.08105759021766E-6));
#13143=CARTESIAN_POINT('Ctrl Pts',(0.203110344361254,-1.14653799330522,
-1.10782444979703E-6));
#13144=CARTESIAN_POINT('Ctrl Pts',(0.204308287281872,-1.15147379958167,
-1.12500597321754E-6));
#13145=CARTESIAN_POINT('Ctrl Pts',(0.205876831658669,-1.15632444796435,
-7.573778542164E-7));
#13146=CARTESIAN_POINT('Ctrl Pts',(0.207807574899602,-1.16104329283393,
-1.57887042599725E-7));
#13147=CARTESIAN_POINT('Ctrl Pts',(0.21096922807971,-1.1687705506961,8.23798139982571E-7));
#13148=CARTESIAN_POINT('Ctrl Pts',(0.215060220496011,-1.17605061753432,
2.67511715935828E-6));
#13149=CARTESIAN_POINT('Ctrl Pts',(0.220020901709485,-1.18268777995331,
1.20301732358232E-6));
#13150=CARTESIAN_POINT('Ctrl Pts',(0.222788929945646,-1.18639127392786,
3.81595076007225E-7));
#13151=CARTESIAN_POINT('Ctrl Pts',(0.225828882930032,-1.18989419630164,
-1.55522758636672E-6));
#13152=CARTESIAN_POINT('Ctrl Pts',(0.229112809647272,-1.19317965616817,
-3.52099818518546E-6));
#13153=CARTESIAN_POINT('Ctrl Pts',(0.234731790749985,-1.1988012605745,-6.88454091865859E-6));
#13154=CARTESIAN_POINT('Ctrl Pts',(0.240999377733319,-1.20372479786492,
-1.00686973618824E-5));
#13155=CARTESIAN_POINT('Ctrl Pts',(0.247759525934523,-1.2078808899968,-1.07387199666626E-5));
#13156=CARTESIAN_POINT('Ctrl Pts',(0.251104201987095,-1.20993717358883,
-1.10702228411842E-5));
#13157=CARTESIAN_POINT('Ctrl Pts',(0.254570062984725,-1.21180502729412,
-1.08478245319173E-5));
#13158=CARTESIAN_POINT('Ctrl Pts',(0.258140701417296,-1.21347208138814,
-1.01264154182862E-5));
#13159=CARTESIAN_POINT('Ctrl Pts',(0.265309933881728,-1.21681924144269,
-8.67794906268977E-6));
#13160=CARTESIAN_POINT('Ctrl Pts',(0.27282354441991,-1.21932394229889,-5.03816435877804E-6));
#13161=CARTESIAN_POINT('Ctrl Pts',(0.280540402387729,-1.22090470300999,
-2.38011023443526E-6));
#13162=CARTESIAN_POINT('Ctrl Pts',(0.284441227387562,-1.22170376798259,
-1.03647996128718E-6));
#13163=CARTESIAN_POINT('Ctrl Pts',(0.288394358015454,-1.22226603782358,
-8.41267709508591E-12));
#13164=CARTESIAN_POINT('Ctrl Pts',(0.292382661757373,-1.22257596919059,
3.10081821330854E-17));
#13165=CARTESIAN_POINT('',(0.9,-1.266106713614,0.));
#13166=CARTESIAN_POINT('Ctrl Pts',(0.29238266175737,-1.22257596919059,3.4274341177698E-16));
#13167=CARTESIAN_POINT('Ctrl Pts',(0.494894519961671,-1.23831317320793,
3.6654050078524E-12));
#13168=CARTESIAN_POINT('Ctrl Pts',(0.697432753591781,-1.25280566766171,
-2.10377631034678E-8));
#13169=CARTESIAN_POINT('Ctrl Pts',(0.900000000000002,-1.266106713614,4.80511808774455E-17));
#13170=CARTESIAN_POINT('',(0.9,1.34328341716202,0.));
#13171=CARTESIAN_POINT('',(3.5,-1.37552980833516,0.));
#13172=CARTESIAN_POINT('Ctrl Pts',(1.10000000028363,-1.27885335028943,-5.13283219638443E-11));
#13173=CARTESIAN_POINT('Ctrl Pts',(1.8994825293422,-1.32827224294784,2.51289069808066E-7));
#13174=CARTESIAN_POINT('Ctrl Pts',(2.69943073922525,-1.35940904940056,2.35357980118634E-7));
#13175=CARTESIAN_POINT('Ctrl Pts',(3.50000000097418,-1.37552980835478,8.59034485311056E-16));
#13176=CARTESIAN_POINT('',(3.5,1.44777777777778,0.));
#13177=CARTESIAN_POINT('',(7.1,-1.35793097395724,0.));
#13178=CARTESIAN_POINT('Ctrl Pts',(3.700000000362,-1.379246395385,-6.25385501848083E-12));
#13179=CARTESIAN_POINT('Ctrl Pts',(4.26467016042339,-1.38886773733237,1.63880713394601E-8));
#13180=CARTESIAN_POINT('Ctrl Pts',(4.82965558050887,-1.39115503781354,-4.12727732537403E-8));
#13181=CARTESIAN_POINT('Ctrl Pts',(5.39500817395676,-1.38725486475042,-3.97626883737645E-8));
#13182=CARTESIAN_POINT('Ctrl Pts',(5.96336684492344,-1.38333395379258,-3.82445741104923E-8));
#13183=CARTESIAN_POINT('Ctrl Pts',(6.53173538886785,-1.37316170188981,3.71969681223073E-9));
#13184=CARTESIAN_POINT('Ctrl Pts',(7.1000000000396,-1.35793097389613,-4.88946831112289E-12));
#13185=CARTESIAN_POINT('',(7.1,1.42555555555556,0.));
#13186=CARTESIAN_POINT('',(10.2,-1.23178301601145,0.));
#13187=CARTESIAN_POINT('',(10.5052647440597,-1.21555035534119,0.));
#13188=CARTESIAN_POINT('Ctrl Pts',(10.2,-1.23178301601145,-4.56855690431079E-17));
#13189=CARTESIAN_POINT('Ctrl Pts',(10.3017652114452,-1.22646242153193,-6.28718440835499E-11));
#13190=CARTESIAN_POINT('Ctrl Pts',(10.4035203469111,-1.22104923788321,1.43982679105611E-13));
#13191=CARTESIAN_POINT('Ctrl Pts',(10.5052647440597,-1.21555035534119,6.44897004721534E-17));
#13192=CARTESIAN_POINT('',(10.5997255308004,-1.11583328740478,1.38777878078145E-17));
#13193=CARTESIAN_POINT('Ctrl Pts',(10.5052647440597,-1.21555035534119,-1.86482773667507E-17));
#13194=CARTESIAN_POINT('Ctrl Pts',(10.5131888530666,-1.21512208850275,-5.60416335832109E-13));
#13195=CARTESIAN_POINT('Ctrl Pts',(10.5210180054001,-1.21372544600509,-1.35972994235015E-6));
#13196=CARTESIAN_POINT('Ctrl Pts',(10.5285917824072,-1.2114444991589,-1.66070161277884E-6));
#13197=CARTESIAN_POINT('Ctrl Pts',(10.5334522234388,-1.20998071066451,-1.8538489757029E-6));
#13198=CARTESIAN_POINT('Ctrl Pts',(10.538207639053,-1.20815156029678,-1.66445033219183E-6));
#13199=CARTESIAN_POINT('Ctrl Pts',(10.542812250732,-1.20596855068549,-1.19054254011085E-6));
#13200=CARTESIAN_POINT('Ctrl Pts',(10.5499808226381,-1.20256998801374,-4.52751316616249E-7));
#13201=CARTESIAN_POINT('Ctrl Pts',(10.5567010840309,-1.19835579238971,1.16775294480959E-6));
#13202=CARTESIAN_POINT('Ctrl Pts',(10.5628099082467,-1.1933896765605,3.12218506849373E-7));
#13203=CARTESIAN_POINT('Ctrl Pts',(10.563392699667,-1.1929159013142,2.30599178383296E-7));
#13204=CARTESIAN_POINT('Ctrl Pts',(10.563969906567,-1.19243524850296,1.23643260424227E-7));
#13205=CARTESIAN_POINT('Ctrl Pts',(10.5645413730323,-1.19194775268147,-1.33988689923433E-8));
#13206=CARTESIAN_POINT('Ctrl Pts',(10.5677990734116,-1.18916873515523,-7.94620907596477E-7));
#13207=CARTESIAN_POINT('Ctrl Pts',(10.5708705204042,-1.18616755700159,-2.52696578471864E-6));
#13208=CARTESIAN_POINT('Ctrl Pts',(10.5737438185805,-1.18296717200411,-4.3349897000341E-6));
#13209=CARTESIAN_POINT('Ctrl Pts',(10.579054042416,-1.17705244973962,-7.67644996655303E-6));
#13210=CARTESIAN_POINT('Ctrl Pts',(10.5836289246435,-1.17052745137283,-1.0999028846932E-5));
#13211=CARTESIAN_POINT('Ctrl Pts',(10.5874112735695,-1.16355342251842,-1.18035167459916E-5));
#13212=CARTESIAN_POINT('Ctrl Pts',(10.5894705469099,-1.15975646143,-1.22415145393192E-5));
#13213=CARTESIAN_POINT('Ctrl Pts',(10.5912942421259,-1.15582570378367,-1.20038889321768E-5));
#13214=CARTESIAN_POINT('Ctrl Pts',(10.5928674986933,-1.15178403025788,-1.11465830745351E-5));
#13215=CARTESIAN_POINT('Ctrl Pts',(10.5957384082276,-1.14440870489779,-9.58215448007377E-6));
#13216=CARTESIAN_POINT('Ctrl Pts',(10.5977463817932,-1.13674651935037,-5.80208140981121E-6));
#13217=CARTESIAN_POINT('Ctrl Pts',(10.5988207707371,-1.12894377506163,-2.8960211281105E-6));
#13218=CARTESIAN_POINT('Ctrl Pts',(10.5994175893465,-1.12460938291963,-1.28171667533415E-6));
#13219=CARTESIAN_POINT('Ctrl Pts',(10.5997255306822,-1.12023121224821,-9.4020583932734E-12));
#13220=CARTESIAN_POINT('Ctrl Pts',(10.5997255308004,-1.11583328740478,-9.97465998686664E-18));
#13221=CARTESIAN_POINT('',(10.5997255308004,1.11583328740478,0.));
#13222=CARTESIAN_POINT('',(10.5997255308004,0.7,0.));
#13223=CARTESIAN_POINT('',(10.5052647440597,1.21555035534119,0.));
#13224=CARTESIAN_POINT('Ctrl Pts',(10.5997255308004,1.11583328740478,8.8037216405823E-17));
#13225=CARTESIAN_POINT('Ctrl Pts',(10.5997255307124,1.12376989384288,-2.22024716398596E-12));
#13226=CARTESIAN_POINT('Ctrl Pts',(10.5987536115518,1.13166401228391,-1.27532141444775E-6));
#13227=CARTESIAN_POINT('Ctrl Pts',(10.5968849989732,1.13935090273995,-1.5236651967046E-6));
#13228=CARTESIAN_POINT('Ctrl Pts',(10.5956849616024,1.14428748291596,-1.68315348385219E-6));
#13229=CARTESIAN_POINT('Ctrl Pts',(10.5941139374364,1.14913880701507,-1.46899737395989E-6));
#13230=CARTESIAN_POINT('Ctrl Pts',(10.5921809408638,1.1538584293407,-9.90118991603547E-7));
#13231=CARTESIAN_POINT('Ctrl Pts',(10.5891742477341,1.16119959911942,-2.45244239835432E-7));
#13232=CARTESIAN_POINT('Ctrl Pts',(10.5853292249979,1.16813727090899,1.33309554558619E-6));
#13233=CARTESIAN_POINT('Ctrl Pts',(10.5807005079991,1.17450509276749,4.08358240744415E-7));
#13234=CARTESIAN_POINT('Ctrl Pts',(10.5802604812716,1.17511044665166,3.20448539159982E-7));
#13235=CARTESIAN_POINT('Ctrl Pts',(10.5798133373602,1.17571063303672,2.07176952714776E-7));
#13236=CARTESIAN_POINT('Ctrl Pts',(10.5793591019426,1.17630549598644,6.38823567561716E-8));
#13237=CARTESIAN_POINT('Ctrl Pts',(10.5767566952267,1.17971358631841,-7.57081408668461E-7));
#13238=CARTESIAN_POINT('Ctrl Pts',(10.5739217504488,1.18294722379721,-2.53660858190298E-6));
#13239=CARTESIAN_POINT('Ctrl Pts',(10.570876618072,1.18599321478588,-4.38998728286835E-6));
#13240=CARTESIAN_POINT('Ctrl Pts',(10.5652565693637,1.19161484813492,-7.81055403847458E-6));
#13241=CARTESIAN_POINT('Ctrl Pts',(10.5589874561388,1.19653507038546,-1.11999964534866E-5));
#13242=CARTESIAN_POINT('Ctrl Pts',(10.5522271124844,1.20068789486255,-1.20263298844839E-5));
#13243=CARTESIAN_POINT('Ctrl Pts',(10.5485500617744,1.20294667739977,-1.24757848359648E-5));
#13244=CARTESIAN_POINT('Ctrl Pts',(10.5447269560479,1.20497781184918,-1.22374322375965E-5));
#13245=CARTESIAN_POINT('Ctrl Pts',(10.5407797717187,1.20676523914267,-1.13674773191707E-5));
#13246=CARTESIAN_POINT('Ctrl Pts',(10.5335711832013,1.210029547771,-9.77871264224002E-6));
#13247=CARTESIAN_POINT('Ctrl Pts',(10.5260296312848,1.21244761587922,-5.9245235663186E-6));
#13248=CARTESIAN_POINT('Ctrl Pts',(10.5182973307397,1.21394093281975,-2.95733858081469E-6));
#13249=CARTESIAN_POINT('Ctrl Pts',(10.514004731837,1.21476995008607,-1.31010113336685E-6));
#13250=CARTESIAN_POINT('Ctrl Pts',(10.5096528988527,1.21531319279956,-7.28166367327128E-12));
#13251=CARTESIAN_POINT('Ctrl Pts',(10.5052647440597,1.21555035534119,-3.31765864780564E-17));
#13252=CARTESIAN_POINT('',(10.2,1.23178301601145,0.));
#13253=CARTESIAN_POINT('Ctrl Pts',(10.5052647440597,1.21555035534119,1.20285454773689E-16));
#13254=CARTESIAN_POINT('Ctrl Pts',(10.4035203468995,1.22104923788384,1.44021921739714E-13));
#13255=CARTESIAN_POINT('Ctrl Pts',(10.3017652114309,1.22646242153268,-6.28696045710378E-11));
#13256=CARTESIAN_POINT('Ctrl Pts',(10.2,1.23178301601145,1.23125603768043E-16));
#13257=CARTESIAN_POINT('',(10.2,-1.30754691548544,0.));
#13258=CARTESIAN_POINT('Origin',(8.8,0.,0.));
#13259=CARTESIAN_POINT('',(8.4,-4.89858719658942E-17,0.));
#13260=CARTESIAN_POINT('Origin',(2.,0.,0.));
#13261=CARTESIAN_POINT('',(1.6,-4.89858719658941E-17,0.7));
#13262=CARTESIAN_POINT('Origin',(2.,0.,0.7));
#13263=CARTESIAN_POINT('',(1.6,-4.89858719658941E-17,0.));
#13264=CARTESIAN_POINT('Origin',(10.2,-1.30754691548544,0.));
#13265=CARTESIAN_POINT('',(10.1999999975107,-1.19856231453552,0.605472757505173));
#13266=CARTESIAN_POINT('Ctrl Pts',(10.2,-1.23178301601145,0.));
#13267=CARTESIAN_POINT('Ctrl Pts',(10.2,-1.22625045235593,0.100869147801815));
#13268=CARTESIAN_POINT('Ctrl Pts',(10.2,-1.22071692450357,0.201739022585575));
#13269=CARTESIAN_POINT('Ctrl Pts',(10.2,-1.2096433936729,0.403562754186249));
#13270=CARTESIAN_POINT('Ctrl Pts',(10.1999999975107,-1.20410330368611,0.50451817268257));
#13271=CARTESIAN_POINT('Ctrl Pts',(10.1999999975107,-1.19856231453552,0.605472757505173));
#13272=CARTESIAN_POINT('',(10.1999999975107,1.19856231453552,0.605472757505173));
#13273=CARTESIAN_POINT('Ctrl Pts',(10.1999999975107,1.19856231453552,0.605472757505173));
#13274=CARTESIAN_POINT('Ctrl Pts',(10.1999999975107,1.20410418062036,0.504502195294633));
#13275=CARTESIAN_POINT('Ctrl Pts',(10.2,1.20964514726505,0.403530798997214));
#13276=CARTESIAN_POINT('Ctrl Pts',(10.2,1.22071867750565,0.201707067365009));
#13277=CARTESIAN_POINT('Ctrl Pts',(10.2,1.22625132869937,0.100853170395858));
#13278=CARTESIAN_POINT('Ctrl Pts',(10.2,1.23178301601145,0.));
#13279=CARTESIAN_POINT('',(10.1999999980542,1.09857320530976,0.7));
#13280=CARTESIAN_POINT('Ctrl Pts',(10.1999999999973,1.09857320510493,0.7));
#13281=CARTESIAN_POINT('Ctrl Pts',(10.2000000008642,1.10649088744708,0.699999999248278));
#13282=CARTESIAN_POINT('Ctrl Pts',(10.1999989363772,1.11434529358656,0.699006164779054));
#13283=CARTESIAN_POINT('Ctrl Pts',(10.1999980093114,1.12199598895487,0.697118997523365));
#13284=CARTESIAN_POINT('Ctrl Pts',(10.1999974900707,1.12628106973794,0.696062013320951));
#13285=CARTESIAN_POINT('Ctrl Pts',(10.1999970168623,1.13050229860485,0.694723760583242));
#13286=CARTESIAN_POINT('Ctrl Pts',(10.199996713894,1.13463332887353,0.693115046692397));
#13287=CARTESIAN_POINT('Ctrl Pts',(10.1999961690675,1.14206214329588,0.690222103243312));
#13288=CARTESIAN_POINT('Ctrl Pts',(10.1999962772589,1.14911941279843,0.686488866209959));
#13289=CARTESIAN_POINT('Ctrl Pts',(10.1999969599022,1.15565885618684,0.681996408643444));
#13290=CARTESIAN_POINT('Ctrl Pts',(10.1999973343062,1.15924549304116,0.679532465931891));
#13291=CARTESIAN_POINT('Ctrl Pts',(10.1999978674396,1.16267609380848,0.676839263748528));
#13292=CARTESIAN_POINT('Ctrl Pts',(10.1999983417863,1.16592263776853,0.673924718551186));
#13293=CARTESIAN_POINT('Ctrl Pts',(10.199998806773,1.16910511991263,0.671067684066867));
#13294=CARTESIAN_POINT('Ctrl Pts',(10.1999992207276,1.17209141256199,0.668015240668471));
#13295=CARTESIAN_POINT('Ctrl Pts',(10.1999992206607,1.17485880184773,0.664778864469812));
#13296=CARTESIAN_POINT('Ctrl Pts',(10.1999992205369,1.17997899231675,0.658790960038769));
#13297=CARTESIAN_POINT('Ctrl Pts',(10.1999979581638,1.18435276586188,0.652174799271591));
#13298=CARTESIAN_POINT('Ctrl Pts',(10.1999975326045,1.18791964688485,0.645095405674036));
#13299=CARTESIAN_POINT('Ctrl Pts',(10.1999974898604,1.18827791229431,0.644384335742179));
#13300=CARTESIAN_POINT('Ctrl Pts',(10.1999974535047,1.18862799840101,0.643668573506599));
#13301=CARTESIAN_POINT('Ctrl Pts',(10.1999974242393,1.18896981696374,0.64294827577739));
#13302=CARTESIAN_POINT('Ctrl Pts',(10.1999971329942,1.1923715530028,0.635779961907205));
#13303=CARTESIAN_POINT('Ctrl Pts',(10.1999977790614,1.19491900203126,0.628247233077589));
#13304=CARTESIAN_POINT('Ctrl Pts',(10.1999987199397,1.19655829940385,0.620518158911201));
#13305=CARTESIAN_POINT('Ctrl Pts',(10.1999993222661,1.19760773597399,0.615570201805241));
#13306=CARTESIAN_POINT('Ctrl Pts',(10.2,1.19828413277105,0.610541112135461));
#13307=CARTESIAN_POINT('Ctrl Pts',(10.2,1.19856231427281,0.60547275750556));
#13308=CARTESIAN_POINT('',(10.2,-1.09857320510402,0.7));
#13309=CARTESIAN_POINT('',(10.2,-0.653773457742722,0.7));
#13310=CARTESIAN_POINT('Ctrl Pts',(10.2,-1.19856231427281,0.60547275750556));
#13311=CARTESIAN_POINT('Ctrl Pts',(10.2,-1.19812809376428,0.613384079828744));
#13312=CARTESIAN_POINT('Ctrl Pts',(10.1999984889428,-1.1967261327477,0.621202329970501));
#13313=CARTESIAN_POINT('Ctrl Pts',(10.1999978161146,-1.19444079525024,0.628767398200536));
#13314=CARTESIAN_POINT('Ctrl Pts',(10.1999974438306,-1.19317629038787,0.632953241898348));
#13315=CARTESIAN_POINT('Ctrl Pts',(10.1999972759003,-1.19164034846853,0.637061602680377));
#13316=CARTESIAN_POINT('Ctrl Pts',(10.1999973648938,-1.18984073583679,0.641063423920242));
#13317=CARTESIAN_POINT('Ctrl Pts',(10.1999975257516,-1.18658789218766,0.648296813248274));
#13318=CARTESIAN_POINT('Ctrl Pts',(10.1999986492083,-1.18251199594868,0.655103972585077));
#13319=CARTESIAN_POINT('Ctrl Pts',(10.1999990866637,-1.1776776067306,0.66132208754656));
#13320=CARTESIAN_POINT('Ctrl Pts',(10.1999991692372,-1.17676507450965,0.662495809810115));
#13321=CARTESIAN_POINT('Ctrl Pts',(10.1999992204458,-1.17582538639523,0.663648473741297));
#13322=CARTESIAN_POINT('Ctrl Pts',(10.1999992199672,-1.17485880188435,0.664778864469789));
#13323=CARTESIAN_POINT('Ctrl Pts',(10.1999992190419,-1.17299032792757,0.666963987046661));
#13324=CARTESIAN_POINT('Ctrl Pts',(10.1999990265713,-1.17102137903347,0.669065925022507));
#13325=CARTESIAN_POINT('Ctrl Pts',(10.1999987631451,-1.16895889720817,0.671081139337088));
#13326=CARTESIAN_POINT('Ctrl Pts',(10.1999980371048,-1.16327440276409,0.676635357771578));
#13327=CARTESIAN_POINT('Ctrl Pts',(10.1999968952367,-1.15694629605269,0.681471105251756));
#13328=CARTESIAN_POINT('Ctrl Pts',(10.1999965193249,-1.15013861030111,0.685534582868085));
#13329=CARTESIAN_POINT('Ctrl Pts',(10.1999962798276,-1.14580136285465,0.688123466749966));
#13330=CARTESIAN_POINT('Ctrl Pts',(10.1999963003895,-1.14126848503633,0.690398200126003));
#13331=CARTESIAN_POINT('Ctrl Pts',(10.1999965837416,-1.13657664085124,0.692335536714198));
#13332=CARTESIAN_POINT('Ctrl Pts',(10.199997026059,-1.12925259320479,0.695359751696499));
#13333=CARTESIAN_POINT('Ctrl Pts',(10.1999981114625,-1.12162598460505,0.697529439192009));
#13334=CARTESIAN_POINT('Ctrl Pts',(10.1999989867727,-1.11384404680861,0.698775198878229));
#13335=CARTESIAN_POINT('Ctrl Pts',(10.1999995533653,-1.10880676031141,0.699581585232154));
#13336=CARTESIAN_POINT('Ctrl Pts',(10.200000000559,-1.10370379302489,0.699999999512891));
#13337=CARTESIAN_POINT('Ctrl Pts',(10.1999999999973,-1.09857320510493,0.7));
#13338=CARTESIAN_POINT('Ctrl Pts',(10.0273290644374,-1.24073895154929,-0.000342977371441382));
#13339=CARTESIAN_POINT('Ctrl Pts',(10.0182194939277,-1.2301570933055,0.201590462913323));
#13340=CARTESIAN_POINT('Ctrl Pts',(10.0091098064739,-1.21957524432673,0.403523898419685));
#13341=CARTESIAN_POINT('Ctrl Pts',(10.,-1.20899340483173,0.605457329065658));
#13342=CARTESIAN_POINT('Ctrl Pts',(9.11786336174441,-1.287320026752,-0.000205293215301774));
#13343=CARTESIAN_POINT('Ctrl Pts',(9.11054075262461,-1.27673792859995,0.201728409731728));
#13344=CARTESIAN_POINT('Ctrl Pts',(9.10321803982027,-1.2661558351744,0.403662109352091));
#13345=CARTESIAN_POINT('Ctrl Pts',(9.09589522044064,-1.25557375159922,0.605595805683776));
#13346=CARTESIAN_POINT('Ctrl Pts',(8.20875307681921,-1.32613868191631,-8.19769783003664E-5));
#13347=CARTESIAN_POINT('Ctrl Pts',(8.20321812688803,-1.31555630757271,0.201851960079368));
#13348=CARTESIAN_POINT('Ctrl Pts',(8.19768309032111,-1.30497393555236,0.403785895133155));
#13349=CARTESIAN_POINT('Ctrl Pts',(8.19214796413157,-1.29439157095064,0.605719828258773));
#13350=CARTESIAN_POINT('Ctrl Pts',(7.29999999999999,-1.35236351479115,1.04083408558608E-17));
#13351=CARTESIAN_POINT('Ctrl Pts',(7.29625341766944,-1.34178092325774,0.201934092022114));
#13352=CARTESIAN_POINT('Ctrl Pts',(7.2925067690755,-1.33119833465137,0.403868182971915));
#13353=CARTESIAN_POINT('Ctrl Pts',(7.28876005303739,-1.32061574904145,0.605802272831199));
#13354=CARTESIAN_POINT('Ctrl Pts',(7.29999999953094,-1.32031613471704,0.605285370449856));
#13355=CARTESIAN_POINT('Ctrl Pts',(8.20058408060299,-1.29406305600824,0.605326635812744));
#13356=CARTESIAN_POINT('Ctrl Pts',(9.10058974048747,-1.25534320916473,0.605388449123016));
#13357=CARTESIAN_POINT('Ctrl Pts',(9.99999999968202,-1.20899340489109,0.605457329065633));
#13358=CARTESIAN_POINT('Ctrl Pts',(10.5052670937641,-1.21555282972197,-4.72190879230918E-5));
#13359=CARTESIAN_POINT('Ctrl Pts',(10.4952228315222,-1.20497561405085,0.201799837144789));
#13360=CARTESIAN_POINT('Ctrl Pts',(10.4851784461209,-1.19439840869387,0.403646887802288));
#13361=CARTESIAN_POINT('Ctrl Pts',(10.4751339353761,-1.18382121389426,0.605493932788863));
#13362=CARTESIAN_POINT('Ctrl Pts',(10.4035069533234,-1.22105168617584,-3.13467776074076E-5));
#13363=CARTESIAN_POINT('Ctrl Pts',(10.3936624949941,-1.21047444506522,0.201815739766394));
#13364=CARTESIAN_POINT('Ctrl Pts',(10.3838179147697,-1.19989721405033,0.403662820908308));
#13365=CARTESIAN_POINT('Ctrl Pts',(10.3739732104882,-1.18931999337004,0.605509896555428));
#13366=CARTESIAN_POINT('Ctrl Pts',(10.3017512542637,-1.22646400658821,-1.55943981238903E-5));
#13367=CARTESIAN_POINT('Ctrl Pts',(10.2921066085356,-1.21588673949083,0.201831522212972));
#13368=CARTESIAN_POINT('Ctrl Pts',(10.2824618422276,-1.20530948226626,0.403678633593635));
#13369=CARTESIAN_POINT('Ctrl Pts',(10.2728169532007,-1.19473223514815,0.605525739654126));
#13370=CARTESIAN_POINT('Ctrl Pts',(10.2,-1.23178301601145,-4.5102810375397E-17));
#13371=CARTESIAN_POINT('Ctrl Pts',(10.1905551755811,-1.22120572247414,0.20184714636246));
#13372=CARTESIAN_POINT('Ctrl Pts',(10.1811102319487,-1.21062843858304,0.403694287664275));
#13373=CARTESIAN_POINT('Ctrl Pts',(10.1716651669877,-1.20005116456574,0.605541423818621));
#13374=CARTESIAN_POINT('',(10.4735630903435,-1.18390659316268,0.605494180667944));
#13375=CARTESIAN_POINT('Ctrl Pts',(10.1999999975038,-1.19856231440453,0.605472757505366));
#13376=CARTESIAN_POINT('Ctrl Pts',(10.2911933328565,-1.19375025772558,0.605479840815741));
#13377=CARTESIAN_POINT('Ctrl Pts',(10.3823809652617,-1.18886335120032,0.605486986548286));
#13378=CARTESIAN_POINT('Ctrl Pts',(10.4735630903435,-1.18390659316268,0.605494180667944));
#13379=CARTESIAN_POINT('Ctrl Pts',(10.4735630903435,-1.18390659316268,0.605494180667945));
#13380=CARTESIAN_POINT('Ctrl Pts',(10.4841302498201,-1.19445434834508,0.403662775875149));
#13381=CARTESIAN_POINT('Ctrl Pts',(10.4946974680575,-1.20500226999407,0.201831382381129));
#13382=CARTESIAN_POINT('Ctrl Pts',(10.5052647440597,-1.21555035534119,-6.86299975183324E-17));
#13383=CARTESIAN_POINT('Ctrl Pts',(10.,-1.10900986674273,0.7));
#13384=CARTESIAN_POINT('Ctrl Pts',(9.09944331332257,-1.15544418981837,0.7));
#13385=CARTESIAN_POINT('Ctrl Pts',(8.1984670949788,-1.19422430779862,0.7));
#13386=CARTESIAN_POINT('Ctrl Pts',(7.29709043526679,-1.22049830417059,0.7));
#13387=CARTESIAN_POINT('Ctrl Pts',(10.0014871213396,-1.13785139984992,0.7));
#13388=CARTESIAN_POINT('Ctrl Pts',(9.10076698492608,-1.18430758604571,0.700000491839571));
#13389=CARTESIAN_POINT('Ctrl Pts',(8.19957769811723,-1.22310890030201,0.699999704549177));
#13390=CARTESIAN_POINT('Ctrl Pts',(7.29793284700475,-1.24939875264889,0.7));
#13391=CARTESIAN_POINT('Ctrl Pts',(10.0040646682326,-1.18784086746588,0.676686753673613));
#13392=CARTESIAN_POINT('Ctrl Pts',(9.10306300621911,-1.23433322993607,0.676664155483858));
#13393=CARTESIAN_POINT('Ctrl Pts',(8.20149954052229,-1.27317186922949,0.676644146017133));
#13394=CARTESIAN_POINT('Ctrl Pts',(7.29939288958795,-1.29948813715084,0.676630595533454));
#13395=CARTESIAN_POINT('Ctrl Pts',(10.0050807923581,-1.20754778500352,0.627085325222079));
#13396=CARTESIAN_POINT('Ctrl Pts',(9.10396596140607,-1.25402923300358,0.627026849623412));
#13397=CARTESIAN_POINT('Ctrl Pts',(8.20225661204673,-1.29285896783792,0.626974637782525));
#13398=CARTESIAN_POINT('Ctrl Pts',(7.29996660609514,-1.31917051289423,0.626939603849942));
#13399=CARTESIAN_POINT('Ctrl Pts',(10.0051416645797,-1.20872835322339,0.605457722909465));
#13400=CARTESIAN_POINT('Ctrl Pts',(9.1040197884667,-1.25519559703033,0.605388684776982));
#13401=CARTESIAN_POINT('Ctrl Pts',(8.20230020786566,-1.29401302889245,0.605326714446839));
#13402=CARTESIAN_POINT('Ctrl Pts',(7.29999999953094,-1.32031613471704,0.605285370449856));
#13403=CARTESIAN_POINT('Ctrl Pts',(10.4681436286308,-1.08420482079362,0.7));
#13404=CARTESIAN_POINT('Ctrl Pts',(10.3770124662346,-1.0891584122264,0.7));
#13405=CARTESIAN_POINT('Ctrl Pts',(10.285877616441,-1.09404209584202,0.7));
#13406=CARTESIAN_POINT('Ctrl Pts',(10.1947388861048,-1.09885088260188,0.7));
#13407=CARTESIAN_POINT('Ctrl Pts',(10.4697107510168,-1.11303515260326,0.7));
#13408=CARTESIAN_POINT('Ctrl Pts',(10.3785648662465,-1.11799094453753,0.700000051218742));
#13409=CARTESIAN_POINT('Ctrl Pts',(10.2874149314686,-1.12287675076168,0.699999949550842));
#13410=CARTESIAN_POINT('Ctrl Pts',(10.196260416419,-1.12768774893097,0.7));
#13411=CARTESIAN_POINT('Ctrl Pts',(10.4724269697127,-1.16300539549315,0.676698381019543));
#13412=CARTESIAN_POINT('Ctrl Pts',(10.3812557252598,-1.16796482352885,0.676696026813929));
#13413=CARTESIAN_POINT('Ctrl Pts',(10.2900793016129,-1.17285439035486,0.676693724638983));
#13414=CARTESIAN_POINT('Ctrl Pts',(10.1988975981852,-1.17766904563614,0.67669140632491));
#13415=CARTESIAN_POINT('Ctrl Pts',(10.4734985149421,-1.18271860027509,0.627116141711795));
#13416=CARTESIAN_POINT('Ctrl Pts',(10.382317043787,-1.18767684023183,0.627110048826767));
#13417=CARTESIAN_POINT('Ctrl Pts',(10.2911301919381,-1.19256517083271,0.627104033151799));
#13418=CARTESIAN_POINT('Ctrl Pts',(10.1999375452555,-1.19737868557977,0.627098033786781));
#13419=CARTESIAN_POINT('Ctrl Pts',(10.4735630903435,-1.18390659316268,0.605494180667944));
#13420=CARTESIAN_POINT('Ctrl Pts',(10.3823809652617,-1.18886335120032,0.605486986548286));
#13421=CARTESIAN_POINT('Ctrl Pts',(10.2911933328565,-1.19375025772558,0.605479840815741));
#13422=CARTESIAN_POINT('Ctrl Pts',(10.1999999975038,-1.19856231440453,0.605472757505366));
#13423=CARTESIAN_POINT('',(10.4681436258201,-1.08420482094639,0.7));
#13424=CARTESIAN_POINT('Ctrl Pts',(10.4681436258201,-1.0842048209464,0.7));
#13425=CARTESIAN_POINT('Ctrl Pts',(10.3787660248044,-1.08906309452597,0.7));
#13426=CARTESIAN_POINT('Ctrl Pts',(10.289384876933,-1.09385412476048,0.7));
#13427=CARTESIAN_POINT('Ctrl Pts',(10.1999999999973,-1.09857320510493,0.7));
#13428=CARTESIAN_POINT('Origin',(10.4681436286308,-1.08420482099672,0.6));
#13429=CARTESIAN_POINT('Origin',(5.4,-8.11656130105013E-18,0.7));
#13430=CARTESIAN_POINT('',(10.4681436286308,1.08420482109828,0.7));
#13431=CARTESIAN_POINT('Ctrl Pts',(10.1999999980461,1.09857320520795,0.7));
#13432=CARTESIAN_POINT('Ctrl Pts',(10.2893848765692,1.09385412478074,0.7));
#13433=CARTESIAN_POINT('Ctrl Pts',(10.3787660260279,1.08906309446088,0.7));
#13434=CARTESIAN_POINT('Ctrl Pts',(10.4681436286308,1.08420482079361,0.7));
#13435=CARTESIAN_POINT('',(10.4681436286308,0.7,0.7));
#13436=CARTESIAN_POINT('Ctrl Pts',(7.3,1.35236351479305,-3.57463069561303E-11));
#13437=CARTESIAN_POINT('Ctrl Pts',(7.29625341766908,1.34178092325856,0.20193409200674));
#13438=CARTESIAN_POINT('Ctrl Pts',(7.29250676907475,1.33119833465113,0.403868182976914));
#13439=CARTESIAN_POINT('Ctrl Pts',(7.28876005303626,1.32061574904014,0.60580227285657));
#13440=CARTESIAN_POINT('Ctrl Pts',(8.20875307682014,1.32613868191819,-8.19770140467192E-5));
#13441=CARTESIAN_POINT('Ctrl Pts',(8.20321812688841,1.31555630757352,0.201851960063995));
#13442=CARTESIAN_POINT('Ctrl Pts',(8.19768309032092,1.3049739355521,0.403785895138154));
#13443=CARTESIAN_POINT('Ctrl Pts',(8.19214796413082,1.29439157094932,0.605719828284144));
#13444=CARTESIAN_POINT('Ctrl Pts',(9.11786336174626,1.28732002675385,-0.000205293251048056));
#13445=CARTESIAN_POINT('Ctrl Pts',(9.11054075262572,1.27673792860073,0.201728409716354));
#13446=CARTESIAN_POINT('Ctrl Pts',(9.10321803982063,1.26615583517412,0.403662109357089));
#13447=CARTESIAN_POINT('Ctrl Pts',(9.09589522044026,1.25557375159787,0.605595805709147));
#13448=CARTESIAN_POINT('Ctrl Pts',(10.0273290644402,1.2407389515511,-0.000342977407187712));
#13449=CARTESIAN_POINT('Ctrl Pts',(10.0182194939295,1.23015709330624,0.201590462897949));
#13450=CARTESIAN_POINT('Ctrl Pts',(10.0091098064748,1.21957524432641,0.403523898424684));
#13451=CARTESIAN_POINT('Ctrl Pts',(10.,1.20899340483035,0.605457329091028));
#13452=CARTESIAN_POINT('Ctrl Pts',(10.2,1.23178301601276,-2.39624899783797E-11));
#13453=CARTESIAN_POINT('Ctrl Pts',(10.1905551755807,1.22120572247504,0.201847146346486));
#13454=CARTESIAN_POINT('Ctrl Pts',(10.1811102319479,1.21062843858352,0.403694287656288));
#13455=CARTESIAN_POINT('Ctrl Pts',(10.1716651669865,1.2000511645658,0.605541423818621));
#13456=CARTESIAN_POINT('Ctrl Pts',(10.3017512542641,1.22646400658951,-1.55944220863836E-5));
#13457=CARTESIAN_POINT('Ctrl Pts',(10.2921066085356,1.2158867394917,0.201831522196997));
#13458=CARTESIAN_POINT('Ctrl Pts',(10.2824618422272,1.20530948226672,0.403678633585648));
#13459=CARTESIAN_POINT('Ctrl Pts',(10.2728169531999,1.19473223514819,0.605525739654127));
#13460=CARTESIAN_POINT('Ctrl Pts',(10.4035069533242,1.22105168617711,-3.13468015701665E-5));
#13461=CARTESIAN_POINT('Ctrl Pts',(10.3936624949945,1.21047444506608,0.201815739750419));
#13462=CARTESIAN_POINT('Ctrl Pts',(10.3838179147698,1.19989721405077,0.40366282090032));
#13463=CARTESIAN_POINT('Ctrl Pts',(10.3739732104878,1.18931999337006,0.605509896555428));
#13464=CARTESIAN_POINT('Ctrl Pts',(10.5052670937653,1.21555282972323,-4.72191118859062E-5));
#13465=CARTESIAN_POINT('Ctrl Pts',(10.495222831523,1.20497561405169,0.201799837128814));
#13466=CARTESIAN_POINT('Ctrl Pts',(10.4851784461213,1.19439840869429,0.403646887794301));
#13467=CARTESIAN_POINT('Ctrl Pts',(10.4751339353761,1.18382121389426,0.605493932788864));
#13468=CARTESIAN_POINT('',(10.4735630903435,1.18390659316268,0.605494180667944));
#13469=CARTESIAN_POINT('Ctrl Pts',(10.5052647440597,1.21555035534119,-4.0462425077159E-16));
#13470=CARTESIAN_POINT('Ctrl Pts',(10.4946974680575,1.20500226999407,0.201831382381129));
#13471=CARTESIAN_POINT('Ctrl Pts',(10.4841302498201,1.19445434834508,0.40366277587515));
#13472=CARTESIAN_POINT('Ctrl Pts',(10.4735630903435,1.18390659316268,0.605494180667945));
#13473=CARTESIAN_POINT('Ctrl Pts',(10.4735630903435,1.18390659316268,0.605494180667944));
#13474=CARTESIAN_POINT('Ctrl Pts',(10.3823809652617,1.18886335120032,0.605486986548286));
#13475=CARTESIAN_POINT('Ctrl Pts',(10.2911933328565,1.19375025772558,0.605479840815741));
#13476=CARTESIAN_POINT('Ctrl Pts',(10.1999999975038,1.19856231440453,0.605472757505366));
#13477=CARTESIAN_POINT('Origin',(7.1,1.42555555555556,0.));
#13478=CARTESIAN_POINT('',(7.0999999994629,-1.32593912634735,0.605276549957215));
#13479=CARTESIAN_POINT('Ctrl Pts',(7.0999999994629,-1.32593912634735,0.605276549957215));
#13480=CARTESIAN_POINT('Ctrl Pts',(7.0999999994629,-1.33126650931098,0.504490734647167));
#13481=CARTESIAN_POINT('Ctrl Pts',(7.1,-1.33659376385849,0.403703958452373));
#13482=CARTESIAN_POINT('Ctrl Pts',(7.1,-1.3472576786761,0.201945747207886));
#13483=CARTESIAN_POINT('Ctrl Pts',(7.1,-1.35259443928223,0.100972400854069));
#13484=CARTESIAN_POINT('Ctrl Pts',(7.1,-1.35793097395724,0.));
#13485=CARTESIAN_POINT('',(7.1,-1.22604182196417,0.7));
#13486=CARTESIAN_POINT('Ctrl Pts',(7.1,-1.22604182196307,0.7));
#13487=CARTESIAN_POINT('Ctrl Pts',(7.1,-1.23395163718705,0.7));
#13488=CARTESIAN_POINT('Ctrl Pts',(7.09999945440688,-1.24179783218049,0.699006056038995));
#13489=CARTESIAN_POINT('Ctrl Pts',(7.09999897931553,-1.2494401870438,0.697119011207626));
#13490=CARTESIAN_POINT('Ctrl Pts',(7.09999871186578,-1.25374240366384,0.696056710937424));
#13491=CARTESIAN_POINT('Ctrl Pts',(7.09999846845149,-1.25798007942473,0.69471034534287));
#13492=CARTESIAN_POINT('Ctrl Pts',(7.09999831430822,-1.26212651101681,0.6930909329195));
#13493=CARTESIAN_POINT('Ctrl Pts',(7.09999803835695,-1.26954956016987,0.690191818885951));
#13494=CARTESIAN_POINT('Ctrl Pts',(7.09999810102228,-1.27659977900265,0.686452252582521));
#13495=CARTESIAN_POINT('Ctrl Pts',(7.09999845706054,-1.28313109767173,0.681953977461377));
#13496=CARTESIAN_POINT('Ctrl Pts',(7.09999865314126,-1.2867280867584,0.679476645189077));
#13497=CARTESIAN_POINT('Ctrl Pts',(7.09999893113315,-1.29016742765117,0.67676830886676));
#13498=CARTESIAN_POINT('Ctrl Pts',(7.09999917787259,-1.2934208019838,0.673837071833988));
#13499=CARTESIAN_POINT('Ctrl Pts',(7.09999941835505,-1.29659167515528,0.670980166997299));
#13500=CARTESIAN_POINT('Ctrl Pts',(7.09999963169439,-1.29956664557352,0.667928795646746));
#13501=CARTESIAN_POINT('Ctrl Pts',(7.09999963110542,-1.30232317314677,0.664694459428825));
#13502=CARTESIAN_POINT('Ctrl Pts',(7.09999963001387,-1.30743194453681,0.658700148145236));
#13503=CARTESIAN_POINT('Ctrl Pts',(7.09999897381858,-1.31179333085743,0.652078782729069));
#13504=CARTESIAN_POINT('Ctrl Pts',(7.09999874753952,-1.31534789998199,0.64499600756552));
#13505=CARTESIAN_POINT('Ctrl Pts',(7.09999872438549,-1.31571162172319,0.644271261689237));
#13506=CARTESIAN_POINT('Ctrl Pts',(7.0999987046402,-1.31606685549941,0.643541664816448));
#13507=CARTESIAN_POINT('Ctrl Pts',(7.09999868869212,-1.31641350913238,0.642807383257706));
#13508=CARTESIAN_POINT('Ctrl Pts',(7.09999853283271,-1.31980133087414,0.635631300872562));
#13509=CARTESIAN_POINT('Ctrl Pts',(7.09999885939544,-1.32233451509485,0.628092322434426));
#13510=CARTESIAN_POINT('Ctrl Pts',(7.09999934101855,-1.32395982399511,0.620358959365968));
#13511=CARTESIAN_POINT('Ctrl Pts',(7.09999964997549,-1.32500244522074,0.615398075635307));
#13512=CARTESIAN_POINT('Ctrl Pts',(7.09999999934316,-1.32567060646853,0.610356529630438));
#13513=CARTESIAN_POINT('Ctrl Pts',(7.09999999981141,-1.32593912630714,0.60527654995744));
#13514=CARTESIAN_POINT('',(7.09999999995537,1.22604182196549,0.7));
#13515=CARTESIAN_POINT('',(7.1,0.712777777777778,0.7));
#13516=CARTESIAN_POINT('',(7.0999999994629,1.32593912634735,0.605276549957215));
#13517=CARTESIAN_POINT('Ctrl Pts',(7.09999999981142,1.32593912630714,0.60527654995744));
#13518=CARTESIAN_POINT('Ctrl Pts',(7.09999999908198,1.32552083177145,0.613190035045322));
#13519=CARTESIAN_POINT('Ctrl Pts',(7.09999922367565,1.32413525001942,0.621012727860624));
#13520=CARTESIAN_POINT('Ctrl Pts',(7.09999888117586,1.32186630199077,0.628584136488803));
#13521=CARTESIAN_POINT('Ctrl Pts',(7.09999868987568,1.32059900146923,0.632813078704371));
#13522=CARTESIAN_POINT('Ctrl Pts',(7.09999860640034,1.3190551184949,0.636963663611311));
#13523=CARTESIAN_POINT('Ctrl Pts',(7.09999865766138,1.31724253497577,0.641005923298765));
#13524=CARTESIAN_POINT('Ctrl Pts',(7.0999987494091,1.31399834762864,0.648240816253195));
#13525=CARTESIAN_POINT('Ctrl Pts',(7.09999933613984,1.30993159792479,0.655050690394837));
#13526=CARTESIAN_POINT('Ctrl Pts',(7.09999956222935,1.30510592187917,0.661272231165006));
#13527=CARTESIAN_POINT('Ctrl Pts',(7.09999960444598,1.30420484616769,0.662433950108221));
#13528=CARTESIAN_POINT('Ctrl Pts',(7.09999963060969,1.30327718139331,0.663575086117144));
#13529=CARTESIAN_POINT('Ctrl Pts',(7.09999963056866,1.30232317316131,0.664694459428815));
#13530=CARTESIAN_POINT('Ctrl Pts',(7.09999963048683,1.30042028596585,0.666927187690779));
#13531=CARTESIAN_POINT('Ctrl Pts',(7.09999952705857,1.29841262431024,0.669073382394206));
#13532=CARTESIAN_POINT('Ctrl Pts',(7.09999938633452,1.29630755303174,0.671129253595323));
#13533=CARTESIAN_POINT('Ctrl Pts',(7.09999900634735,1.29062337821964,0.676680576924663));
#13534=CARTESIAN_POINT('Ctrl Pts',(7.09999841760642,1.2842958957007,0.681513596217188));
#13535=CARTESIAN_POINT('Ctrl Pts',(7.0999982224057,1.2774887935492,0.68557385059291));
#13536=CARTESIAN_POINT('Ctrl Pts',(7.09999809840912,1.27316474526651,0.688153029745784));
#13537=CARTESIAN_POINT('Ctrl Pts',(7.09999810738417,1.26864620899217,0.690419707112974));
#13538=CARTESIAN_POINT('Ctrl Pts',(7.09999825155258,1.26396949224645,0.69235064530212));
#13539=CARTESIAN_POINT('Ctrl Pts',(7.09999847710269,1.25665281355793,0.695371579659609));
#13540=CARTESIAN_POINT('Ctrl Pts',(7.09999903441007,1.2490339950321,0.697538299034574));
#13541=CARTESIAN_POINT('Ctrl Pts',(7.09999948258254,1.24125996729125,0.698781081437474));
#13542=CARTESIAN_POINT('Ctrl Pts',(7.09999977198436,1.23623998534067,0.699583592753232));
#13543=CARTESIAN_POINT('Ctrl Pts',(7.1,1.23115469319345,0.7));
#13544=CARTESIAN_POINT('Ctrl Pts',(7.1,1.22604182196307,0.7));
#13545=CARTESIAN_POINT('Ctrl Pts',(7.1,1.35793097395724,0.));
#13546=CARTESIAN_POINT('Ctrl Pts',(7.1,1.35259441576718,0.100972845781549));
#13547=CARTESIAN_POINT('Ctrl Pts',(7.1,1.34725763161617,0.201946637598055));
#13548=CARTESIAN_POINT('Ctrl Pts',(7.1,1.33659371676552,0.403704849408333));
#13549=CARTESIAN_POINT('Ctrl Pts',(7.0999999994629,1.33126648576411,0.504491180117376));
#13550=CARTESIAN_POINT('Ctrl Pts',(7.0999999994629,1.32593912634735,0.605276549957215));
#13551=CARTESIAN_POINT('Ctrl Pts',(7.11011156210589,-1.35766432821499,-9.27062925672982E-5));
#13552=CARTESIAN_POINT('Ctrl Pts',(7.10674110347764,-1.34708925835705,0.201697046690488));
#13553=CARTESIAN_POINT('Ctrl Pts',(7.10337058314201,-1.33651419103807,0.403486798779133));
#13554=CARTESIAN_POINT('Ctrl Pts',(7.09999999999996,-1.32593912631822,0.605276549958221));
#13555=CARTESIAN_POINT('Ctrl Pts',(5.9694837631095,-1.38835096090528,2.80675674898241E-6));
#13556=CARTESIAN_POINT('Ctrl Pts',(5.96835662351021,-1.37777563343505,0.201792740207853));
#13557=CARTESIAN_POINT('Ctrl Pts',(5.96722945517891,-1.3672003004237,0.40358267322573));
#13558=CARTESIAN_POINT('Ctrl Pts',(5.96610224583462,-1.35662497356325,0.605372606931572));
#13559=CARTESIAN_POINT('Ctrl Pts',(4.8294200007394,-1.39866452387306,3.01102374082134E-5));
#13560=CARTESIAN_POINT('Ctrl Pts',(4.83053730380309,-1.38808904115766,0.201820093264151));
#13561=CARTESIAN_POINT('Ctrl Pts',(4.83165461298617,-1.3775135517806,0.403610075973038));
#13562=CARTESIAN_POINT('Ctrl Pts',(4.83277191472125,-1.36693806692183,0.605400059795761));
#13563=CARTESIAN_POINT('Ctrl Pts',(3.68991216363982,-1.37907703205181,-6.2684699445455E-5));
#13564=CARTESIAN_POINT('Ctrl Pts',(3.69327498756969,-1.36850179198701,0.201727122618256));
#13565=CARTESIAN_POINT('Ctrl Pts',(3.69663785098144,-1.3579265529724,0.403516929334346));
#13566=CARTESIAN_POINT('Ctrl Pts',(3.70000075457889,-1.34735131503281,0.605306735438421));
#13567=CARTESIAN_POINT('Ctrl Pts',(3.69999999992215,-1.34735368792773,0.6052614572053));
#13568=CARTESIAN_POINT('Ctrl Pts',(4.83355316856959,-1.366961322855,0.605214762857233));
#13569=CARTESIAN_POINT('Ctrl Pts',(5.96724522208681,-1.35660163688233,0.605228569880684));
#13570=CARTESIAN_POINT('Ctrl Pts',(7.09999999927392,-1.32593912632169,0.605276549957417));
#13571=CARTESIAN_POINT('Ctrl Pts',(7.1,-1.22604182196307,0.7));
#13572=CARTESIAN_POINT('Ctrl Pts',(5.96696284938742,-1.25674179781664,0.7));
#13573=CARTESIAN_POINT('Ctrl Pts',(4.83327074934872,-1.26710800714677,0.7));
#13574=CARTESIAN_POINT('Ctrl Pts',(3.7,-1.24747724070879,0.7));
#13575=CARTESIAN_POINT('Ctrl Pts',(7.10078315634008,-1.25494559805327,0.7));
#13576=CARTESIAN_POINT('Ctrl Pts',(5.96739926106349,-1.28566432005869,0.700000343763215));
#13577=CARTESIAN_POINT('Ctrl Pts',(4.83328164159484,-1.29603890521481,0.700000334703603));
#13578=CARTESIAN_POINT('Ctrl Pts',(3.69949916377151,-1.27639017438114,0.7));
#13579=CARTESIAN_POINT('Ctrl Pts',(7.10214055788579,-1.30504291366416,0.676629771601708));
#13580=CARTESIAN_POINT('Ctrl Pts',(5.96815960929481,-1.33579288254824,0.676614006760374));
#13581=CARTESIAN_POINT('Ctrl Pts',(4.83329467960724,-1.3461818279488,0.676609489640654));
#13582=CARTESIAN_POINT('Ctrl Pts',(3.69863109538965,-1.3265031696486,0.676624836591801));
#13583=CARTESIAN_POINT('Ctrl Pts',(7.10267376869946,-1.32472200604796,0.626932241521275));
#13584=CARTESIAN_POINT('Ctrl Pts',(5.9684558952243,-1.35546668061705,0.626891484245174));
#13585=CARTESIAN_POINT('Ctrl Pts',(4.83330292199863,-1.36585610284781,0.626879766983475));
#13586=CARTESIAN_POINT('Ctrl Pts',(3.69829020046733,-1.34618280086838,0.626919440930842));
#13587=CARTESIAN_POINT('Ctrl Pts',(7.10270476209941,-1.32586587253612,0.605276664588022));
#13588=CARTESIAN_POINT('Ctrl Pts',(5.96847377630401,-1.35660073810322,0.605228567467576));
#13589=CARTESIAN_POINT('Ctrl Pts',(4.8333022084086,-1.36698748587873,0.605214711607465));
#13590=CARTESIAN_POINT('Ctrl Pts',(3.69827043673666,-1.34732374755196,0.60526152849799));
#13591=CARTESIAN_POINT('Ctrl Pts',(7.1,-1.22604182196307,0.7));
#13592=CARTESIAN_POINT('Ctrl Pts',(5.96696284938742,-1.25674179781664,0.7));
#13593=CARTESIAN_POINT('Ctrl Pts',(4.83327074934872,-1.26710800714677,0.7));
#13594=CARTESIAN_POINT('Ctrl Pts',(3.7,-1.24747724070879,0.7));
#13595=CARTESIAN_POINT('Origin',(5.4,-8.11656130105013E-18,0.7));
#13596=CARTESIAN_POINT('Ctrl Pts',(3.7,1.24747724070879,0.7));
#13597=CARTESIAN_POINT('Ctrl Pts',(4.83327074934871,1.26710800714677,0.7));
#13598=CARTESIAN_POINT('Ctrl Pts',(5.96696284938742,1.25674179781664,0.7));
#13599=CARTESIAN_POINT('Ctrl Pts',(7.1,1.22604182196307,0.7));
#13600=CARTESIAN_POINT('Ctrl Pts',(3.7,1.24747724070879,0.7));
#13601=CARTESIAN_POINT('Ctrl Pts',(4.83327074934871,1.26710800714677,0.7));
#13602=CARTESIAN_POINT('Ctrl Pts',(5.96696284938742,1.25674179781664,0.7));
#13603=CARTESIAN_POINT('Ctrl Pts',(7.1,1.22604182196307,0.7));
#13604=CARTESIAN_POINT('Ctrl Pts',(3.69949916377151,1.27639017438114,0.7));
#13605=CARTESIAN_POINT('Ctrl Pts',(4.83328164159484,1.29603890521481,0.700000334703603));
#13606=CARTESIAN_POINT('Ctrl Pts',(5.96739926106349,1.28566432005869,0.700000343763215));
#13607=CARTESIAN_POINT('Ctrl Pts',(7.10078315634008,1.25494559805327,0.7));
#13608=CARTESIAN_POINT('Ctrl Pts',(3.69863109538965,1.3265031696486,0.676624836591801));
#13609=CARTESIAN_POINT('Ctrl Pts',(4.83329467960724,1.3461818279488,0.676609489640654));
#13610=CARTESIAN_POINT('Ctrl Pts',(5.9681596092948,1.33579288254824,0.676614006760374));
#13611=CARTESIAN_POINT('Ctrl Pts',(7.10214055788579,1.30504291366416,0.676629771601707));
#13612=CARTESIAN_POINT('Ctrl Pts',(3.69829020046733,1.34618280086838,0.626919440930842));
#13613=CARTESIAN_POINT('Ctrl Pts',(4.83330292199863,1.36585610284781,0.626879766983475));
#13614=CARTESIAN_POINT('Ctrl Pts',(5.9684558952243,1.35546668061705,0.626891484245174));
#13615=CARTESIAN_POINT('Ctrl Pts',(7.10267376869946,1.32472200604796,0.626932241521275));
#13616=CARTESIAN_POINT('Ctrl Pts',(3.69827043673666,1.34732374755196,0.60526152849799));
#13617=CARTESIAN_POINT('Ctrl Pts',(4.83330220840859,1.36698748587873,0.605214711607465));
#13618=CARTESIAN_POINT('Ctrl Pts',(5.96847377630401,1.35660073810322,0.605228567467576));
#13619=CARTESIAN_POINT('Ctrl Pts',(7.10270476209941,1.32586587253612,0.605276664588022));
#13620=CARTESIAN_POINT('Ctrl Pts',(7.09999999927392,1.32593912632169,0.605276549957417));
#13621=CARTESIAN_POINT('Ctrl Pts',(5.96724522208681,1.35660163688233,0.605228569880684));
#13622=CARTESIAN_POINT('Ctrl Pts',(4.83355316856959,1.366961322855,0.605214762857233));
#13623=CARTESIAN_POINT('Ctrl Pts',(3.69999999992215,1.34735368792773,0.6052614572053));
#13624=CARTESIAN_POINT('Ctrl Pts',(3.68991216360307,1.37907703216746,-6.26869063400631E-5));
#13625=CARTESIAN_POINT('Ctrl Pts',(3.6932749875452,1.36850179206412,0.201727121146993));
#13626=CARTESIAN_POINT('Ctrl Pts',(3.69663785096921,1.35792655301095,0.403516928598715));
#13627=CARTESIAN_POINT('Ctrl Pts',(3.70000075457892,1.34735131503281,0.605306735438421));
#13628=CARTESIAN_POINT('Ctrl Pts',(4.8294200007272,1.39866452398872,3.01080305115927E-5));
#13629=CARTESIAN_POINT('Ctrl Pts',(4.83053730379496,1.38808904123477,0.201820091792887));
#13630=CARTESIAN_POINT('Ctrl Pts',(4.83165461298211,1.37751355181915,0.403610075237406));
#13631=CARTESIAN_POINT('Ctrl Pts',(4.83277191472127,1.36693806692183,0.605400059795761));
#13632=CARTESIAN_POINT('Ctrl Pts',(5.96948376312183,1.38835096102094,2.80454985295556E-6));
#13633=CARTESIAN_POINT('Ctrl Pts',(5.96835662351844,1.37777563351215,0.201792738736588));
#13634=CARTESIAN_POINT('Ctrl Pts',(5.96722945518303,1.36720030046225,0.403582672490098));
#13635=CARTESIAN_POINT('Ctrl Pts',(5.96610224583462,1.35662497356325,0.605372606931572));
#13636=CARTESIAN_POINT('Ctrl Pts',(7.11011156214274,1.35766432833065,-9.27084994613511E-5));
#13637=CARTESIAN_POINT('Ctrl Pts',(7.10674110350221,1.34708925843416,0.201697045219225));
#13638=CARTESIAN_POINT('Ctrl Pts',(7.10337058315429,1.33651419107662,0.403486798043502));
#13639=CARTESIAN_POINT('Ctrl Pts',(7.09999999999996,1.32593912631822,0.605276549958221));
#13640=CARTESIAN_POINT('Origin',(3.5,1.44777777777778,0.));
#13641=CARTESIAN_POINT('',(3.5,-1.34358136363184,0.605270327458634));
#13642=CARTESIAN_POINT('Ctrl Pts',(3.5,-1.34358136363184,0.605270327458634));
#13643=CARTESIAN_POINT('Ctrl Pts',(3.5,-1.34890136370362,0.504489156176152));
#13644=CARTESIAN_POINT('Ctrl Pts',(3.5,-1.35422123464986,0.403706701640381));
#13645=CARTESIAN_POINT('Ctrl Pts',(3.5,-1.3648706701715,0.201950780690867));
#13646=CARTESIAN_POINT('Ctrl Pts',(3.5,-1.3702003690246,0.100974756199658));
#13647=CARTESIAN_POINT('Ctrl Pts',(3.5,-1.37552980833516,0.));
#13648=CARTESIAN_POINT('',(3.5,-1.24369946473884,0.7));
#13649=CARTESIAN_POINT('Ctrl Pts',(3.49999999991873,-1.24369946470729,0.7));
#13650=CARTESIAN_POINT('Ctrl Pts',(3.49999999896975,-1.25160831520001,0.699999999810925));
#13651=CARTESIAN_POINT('Ctrl Pts',(3.50000040534574,-1.25945374057332,0.69900619751828));
#13652=CARTESIAN_POINT('Ctrl Pts',(3.50000075715473,-1.26709539726361,0.697119355224275));
#13653=CARTESIAN_POINT('Ctrl Pts',(3.5000009551612,-1.27139630362835,0.696057395447694));
#13654=CARTESIAN_POINT('Ctrl Pts',(3.50000113454144,-1.27563271975905,0.694711510656402));
#13655=CARTESIAN_POINT('Ctrl Pts',(3.50000124621709,-1.27977793997275,0.693092697679401));
#13656=CARTESIAN_POINT('Ctrl Pts',(3.50000144618968,-1.28720060051191,0.690193961644836));
#13657=CARTESIAN_POINT('Ctrl Pts',(3.50000138985083,-1.29425038514255,0.686454755369034));
#13658=CARTESIAN_POINT('Ctrl Pts',(3.5000011147959,-1.30078112659466,0.681956784255818));
#13659=CARTESIAN_POINT('Ctrl Pts',(3.50000096334461,-1.30437709646577,0.679480102439082));
#13660=CARTESIAN_POINT('Ctrl Pts',(3.50000075087427,-1.30781543681835,0.676772489296601));
#13661=CARTESIAN_POINT('Ctrl Pts',(3.50000056308077,-1.31106783354026,0.67384203444854));
#13662=CARTESIAN_POINT('Ctrl Pts',(3.50000037990614,-1.31424023611357,0.670983655445047));
#13663=CARTESIAN_POINT('Ctrl Pts',(3.50000021841608,-1.31721646102264,0.667930553458483));
#13664=CARTESIAN_POINT('Ctrl Pts',(3.50000022028926,-1.3199739184757,0.664694242102541));
#13665=CARTESIAN_POINT('Ctrl Pts',(3.50000022375892,-1.32508151834405,0.658699667848218));
#13666=CARTESIAN_POINT('Ctrl Pts',(3.50000072745304,-1.32944146850927,0.652077914129702));
#13667=CARTESIAN_POINT('Ctrl Pts',(3.50000090782832,-1.33299465793893,0.64499486611401));
#13668=CARTESIAN_POINT('Ctrl Pts',(3.50000092626355,-1.33335781125732,0.644270944003422));
#13669=CARTESIAN_POINT('Ctrl Pts',(3.50000094214549,-1.33371249714824,0.643542183465449));
#13670=CARTESIAN_POINT('Ctrl Pts',(3.5000009551778,-1.33405862411533,0.642808750463418));
#13671=CARTESIAN_POINT('Ctrl Pts',(3.50000108270827,-1.3374457225345,0.635631587173848));
#13672=CARTESIAN_POINT('Ctrl Pts',(3.5000008470667,-1.33997810357527,0.628091493562486));
#13673=CARTESIAN_POINT('Ctrl Pts',(3.50000049017339,-1.34160279315579,0.620357239364781));
#13674=CARTESIAN_POINT('Ctrl Pts',(3.50000026118253,-1.3426452308862,0.615394766232079));
#13675=CARTESIAN_POINT('Ctrl Pts',(3.5,-1.34331313055125,0.610351689051435));
#13676=CARTESIAN_POINT('Ctrl Pts',(3.5,-1.34358136363184,0.605270327458634));
#13677=CARTESIAN_POINT('',(3.5,0.723888888888889,0.7));
#13678=CARTESIAN_POINT('Ctrl Pts',(3.5,1.37552980833516,0.));
#13679=CARTESIAN_POINT('Ctrl Pts',(3.5,1.37020035376703,0.10097504527886));
#13680=CARTESIAN_POINT('Ctrl Pts',(3.5,1.36487063968137,0.201951358354439));
#13681=CARTESIAN_POINT('Ctrl Pts',(3.5,1.35422120417274,0.403707279015233));
#13682=CARTESIAN_POINT('Ctrl Pts',(3.5,1.34890134846466,0.504489444860456));
#13683=CARTESIAN_POINT('Ctrl Pts',(3.5,1.34358136363184,0.605270327458635));
#13684=CARTESIAN_POINT('Ctrl Pts',(3.50000000097418,-1.37552980835478,3.46944695195361E-18));
#13685=CARTESIAN_POINT('Ctrl Pts',(3.50374047168104,-1.36494504174376,0.201972406882836));
#13686=CARTESIAN_POINT('Ctrl Pts',(3.50748098869546,-1.35436027657305,0.403944812985359));
#13687=CARTESIAN_POINT('Ctrl Pts',(3.51122155284351,-1.34377551287676,0.605917218294091));
#13688=CARTESIAN_POINT('Ctrl Pts',(2.69119625874569,-1.35924722858667,-7.54309614812119E-5));
#13689=CARTESIAN_POINT('Ctrl Pts',(2.69653217397324,-1.34866266892899,0.20189683354744));
#13690=CARTESIAN_POINT('Ctrl Pts',(2.70186816749714,-1.3380781117335,0.403869096002786));
#13691=CARTESIAN_POINT('Ctrl Pts',(2.7072042346663,-1.32749355863083,0.605841357314298));
#13692=CARTESIAN_POINT('Ctrl Pts',(1.88267190563219,-1.32763345268679,-0.000212792412547521));
#13693=CARTESIAN_POINT('Ctrl Pts',(1.88960380459144,-1.31704931403188,0.201759213581099));
#13694=CARTESIAN_POINT('Ctrl Pts',(1.89653581411498,-1.30646518166523,0.403731216009517));
#13695=CARTESIAN_POINT('Ctrl Pts',(1.90346792975642,-1.29588105699583,0.605703215867581));
#13696=CARTESIAN_POINT('Ctrl Pts',(1.07441451989529,-1.27728918272486,-0.000429194541766893));
#13697=CARTESIAN_POINT('Ctrl Pts',(1.08294287068452,-1.26670581246828,0.201542410257184));
#13698=CARTESIAN_POINT('Ctrl Pts',(1.09147136321593,-1.25612245578053,0.403514009799157));
#13699=CARTESIAN_POINT('Ctrl Pts',(1.09999999999989,-1.24553911298205,0.605485603995245));
#13700=CARTESIAN_POINT('Ctrl Pts',(1.09999999916631,-1.24553911263844,0.605485603997431));
#13701=CARTESIAN_POINT('Ctrl Pts',(1.89930203168262,-1.29563783986497,0.605377360150118));
#13702=CARTESIAN_POINT('Ctrl Pts',(2.69958486793449,-1.32722445934619,0.605308375488923));
#13703=CARTESIAN_POINT('Ctrl Pts',(3.5,-1.34358136363184,0.605270327458634));
#13704=CARTESIAN_POINT('Ctrl Pts',(3.50204003610941,-1.24374118183538,0.7));
#13705=CARTESIAN_POINT('Ctrl Pts',(2.70080437300401,-1.2273695200909,0.7));
#13706=CARTESIAN_POINT('Ctrl Pts',(1.89984199608574,-1.1957170361627,0.7));
#13707=CARTESIAN_POINT('Ctrl Pts',(1.1,-1.14549341399196,0.7));
#13708=CARTESIAN_POINT('Ctrl Pts',(3.50144932661635,-1.27265074030048,0.7));
#13709=CARTESIAN_POINT('Ctrl Pts',(2.6998452019678,-1.25626413437997,0.699999727319846));
#13710=CARTESIAN_POINT('Ctrl Pts',(1.89847848223078,-1.22458382597074,0.70000077422621));
#13711=CARTESIAN_POINT('Ctrl Pts',(1.09819048660397,-1.17431102498992,0.7));
#13712=CARTESIAN_POINT('Ctrl Pts',(3.50042536655637,-1.322763754511,0.676632802377821));
#13713=CARTESIAN_POINT('Ctrl Pts',(2.69818680938114,-1.3063522351595,0.67664530655333));
#13714=CARTESIAN_POINT('Ctrl Pts',(1.89610976425884,-1.27462253270773,0.67666760713801));
#13715=CARTESIAN_POINT('Ctrl Pts',(1.09505363188407,-1.22426736091617,0.676703190608825));
#13716=CARTESIAN_POINT('Ctrl Pts',(3.50002334924346,-1.34243864233338,0.626926882269943));
#13717=CARTESIAN_POINT('Ctrl Pts',(2.6975332861013,-1.32603127467068,0.626959208652505));
#13718=CARTESIAN_POINT('Ctrl Pts',(1.89518106151152,-1.29430885982199,0.62701751976321));
#13719=CARTESIAN_POINT('Ctrl Pts',(1.09381704710221,-1.24396073223232,0.627109609335854));
#13720=CARTESIAN_POINT('Ctrl Pts',(3.5,-1.34358136363184,0.605270327458634));
#13721=CARTESIAN_POINT('Ctrl Pts',(2.69749615303,-1.32718177535833,0.605308474776761));
#13722=CARTESIAN_POINT('Ctrl Pts',(1.89512529323683,-1.29547288309274,0.605377720397184));
#13723=CARTESIAN_POINT('Ctrl Pts',(1.09374258853658,-1.24514653057163,0.605486452199395));
#13724=CARTESIAN_POINT('Ctrl Pts',(3.49999999991875,-1.24369946470729,0.7));
#13725=CARTESIAN_POINT('Ctrl Pts',(3.26917843083003,-1.23897560807887,0.7));
#13726=CARTESIAN_POINT('Ctrl Pts',(3.03837960179139,-1.23298334389983,0.7));
#13727=CARTESIAN_POINT('Ctrl Pts',(2.80762376541487,-1.22564400623233,0.7));
#13728=CARTESIAN_POINT('Ctrl Pts',(2.57739190516312,-1.2178709162388,0.7));
#13729=CARTESIAN_POINT('Ctrl Pts',(2.08463535466707,-1.20026407570248,0.7));
#13730=CARTESIAN_POINT('Ctrl Pts',(1.59210562457525,-1.17639367564078,0.7));
#13731=CARTESIAN_POINT('Ctrl Pts',(1.1,-1.14549341399196,0.7));
#13732=CARTESIAN_POINT('Origin',(5.4,-8.11656130105013E-18,0.7));
#13733=CARTESIAN_POINT('Ctrl Pts',(1.0744145198953,1.27728918272486,-0.000429194541767127));
#13734=CARTESIAN_POINT('Ctrl Pts',(1.08294287068452,1.26670581246828,0.201542410257184));
#13735=CARTESIAN_POINT('Ctrl Pts',(1.09147136321593,1.25612245578053,0.403514009799157));
#13736=CARTESIAN_POINT('Ctrl Pts',(1.0999999999999,1.24553911298205,0.605485603995245));
#13737=CARTESIAN_POINT('Ctrl Pts',(1.88267190563235,1.3276334526868,-0.000212792412547728));
#13738=CARTESIAN_POINT('Ctrl Pts',(1.8896038045916,1.31704931403189,0.201759213581098));
#13739=CARTESIAN_POINT('Ctrl Pts',(1.89653581411514,1.30646518166524,0.403731216009517));
#13740=CARTESIAN_POINT('Ctrl Pts',(1.90346792975658,1.29588105699584,0.605703215867581));
#13741=CARTESIAN_POINT('Ctrl Pts',(2.69119625874601,1.35924722858668,-7.54309614812134E-5));
#13742=CARTESIAN_POINT('Ctrl Pts',(2.69653217397356,1.348662668929,0.201896833547441));
#13743=CARTESIAN_POINT('Ctrl Pts',(2.70186816749745,1.33807811173351,0.403869096002786));
#13744=CARTESIAN_POINT('Ctrl Pts',(2.70720423466661,1.32749355863085,0.605841357314298));
#13745=CARTESIAN_POINT('Ctrl Pts',(3.50000000097466,1.37552980835479,-3.81639164714898E-17));
#13746=CARTESIAN_POINT('Ctrl Pts',(3.50374047168151,1.36494504174377,0.201972406882836));
#13747=CARTESIAN_POINT('Ctrl Pts',(3.50748098869594,1.35436027657306,0.403944812985359));
#13748=CARTESIAN_POINT('Ctrl Pts',(3.51122155284398,1.34377551287677,0.605917218294091));
#13749=CARTESIAN_POINT('Origin',(0.9,1.34328341716202,0.));
#13750=CARTESIAN_POINT('',(0.9,-1.23261418131727,0.605513513251856));
#13751=CARTESIAN_POINT('Ctrl Pts',(0.9,-1.23261418131727,0.605513513251856));
#13752=CARTESIAN_POINT('Ctrl Pts',(0.9,-1.23820195798151,0.504544236118289));
#13753=CARTESIAN_POINT('Ctrl Pts',(0.9,-1.24378834611607,0.403573587101897));
#13754=CARTESIAN_POINT('Ctrl Pts',(0.9,-1.25495246062481,0.201736610752668));
#13755=CARTESIAN_POINT('Ctrl Pts',(0.9,-1.26053033259331,0.100867703930409));
#13756=CARTESIAN_POINT('Ctrl Pts',(0.9,-1.266106713614,0.));
#13757=CARTESIAN_POINT('',(0.9,-1.13254484134404,0.7));
#13758=CARTESIAN_POINT('Ctrl Pts',(0.899999999937205,-1.13254484130906,
0.7));
#13759=CARTESIAN_POINT('Ctrl Pts',(0.899999996287105,-1.14047016437301,
0.699999998205918));
#13760=CARTESIAN_POINT('Ctrl Pts',(0.900001280561548,-1.14833327216777,
0.699006663725481));
#13761=CARTESIAN_POINT('Ctrl Pts',(0.900002371513522,-1.15599299513142,
0.697119896446058));
#13762=CARTESIAN_POINT('Ctrl Pts',(0.900002982478546,-1.16028266409831,
0.696063251566776));
#13763=CARTESIAN_POINT('Ctrl Pts',(0.900003528700818,-1.16450859688491,
0.694725368779139));
#13764=CARTESIAN_POINT('Ctrl Pts',(0.900003857331964,-1.16864431737637,
0.693116947675672));
#13765=CARTESIAN_POINT('Ctrl Pts',(0.900004447924614,-1.17607674172948,
0.690226407030055));
#13766=CARTESIAN_POINT('Ctrl Pts',(0.900004211500339,-1.18313828052408,
0.686496282267003));
#13767=CARTESIAN_POINT('Ctrl Pts',(0.900003280035406,-1.18968205680082,
0.682006679400108));
#13768=CARTESIAN_POINT('Ctrl Pts',(0.900002768383153,-1.19327654302499,
0.679540547464272));
#13769=CARTESIAN_POINT('Ctrl Pts',(0.900002064672634,-1.19671453445753,
0.676844382327844));
#13770=CARTESIAN_POINT('Ctrl Pts',(0.900001450170085,-1.19996775918788,
0.673925988054463));
#13771=CARTESIAN_POINT('Ctrl Pts',(0.900000850201302,-1.20314404102283,
0.67107661751105));
#13772=CARTESIAN_POINT('Ctrl Pts',(0.900000329673364,-1.20612495630093,
0.668032594545539));
#13773=CARTESIAN_POINT('Ctrl Pts',(0.900000346081477,-1.20888784276431,
0.664805176146368));
#13774=CARTESIAN_POINT('Ctrl Pts',(0.900000376514472,-1.21401231436848,
0.658819112599938));
#13775=CARTESIAN_POINT('Ctrl Pts',(0.900002057232535,-1.21838968018573,
0.652203523053766));
#13776=CARTESIAN_POINT('Ctrl Pts',(0.900002698394847,-1.22195969054856,
0.645123732731769));
#13777=CARTESIAN_POINT('Ctrl Pts',(0.900002763240662,-1.22232075393107,
0.644407697543824));
#13778=CARTESIAN_POINT('Ctrl Pts',(0.90000282009371,-1.22267351953901,0.643686895083047));
#13779=CARTESIAN_POINT('Ctrl Pts',(0.900002868017411,-1.22301789747605,
0.642961485862499));
#13780=CARTESIAN_POINT('Ctrl Pts',(0.900003341628975,-1.22642125256928,
0.635792544708285));
#13781=CARTESIAN_POINT('Ctrl Pts',(0.900002645022176,-1.22896979279554,
0.628258742918086));
#13782=CARTESIAN_POINT('Ctrl Pts',(0.900001532827652,-1.23061007098772,
0.6205286650049));
#13783=CARTESIAN_POINT('Ctrl Pts',(0.900000822323555,-1.23165793118585,
0.61559045329652));
#13784=CARTESIAN_POINT('Ctrl Pts',(0.900000000000001,-1.23233426661673,
0.610571479357261));
#13785=CARTESIAN_POINT('Ctrl Pts',(0.900000000000001,-1.23261418131727,
0.605513513251856));
#13786=CARTESIAN_POINT('',(0.9,1.13254484134404,0.7));
#13787=CARTESIAN_POINT('',(0.9,0.671641708581009,0.7));
#13788=CARTESIAN_POINT('',(0.9,1.23261418131727,0.605513513251856));
#13789=CARTESIAN_POINT('Ctrl Pts',(0.9,1.23261418131727,0.605513513251856));
#13790=CARTESIAN_POINT('Ctrl Pts',(0.9,1.23217633603244,0.613425232807268));
#13791=CARTESIAN_POINT('Ctrl Pts',(0.900001832787994,1.23077105609892,0.621244170085157));
#13792=CARTESIAN_POINT('Ctrl Pts',(0.900002580745575,1.22848219166492,0.628809599741497));
#13793=CARTESIAN_POINT('Ctrl Pts',(0.900002993068559,1.22722042035689,0.632980157827643));
#13794=CARTESIAN_POINT('Ctrl Pts',(0.90000314174678,1.22568915198244,0.637073706995481));
#13795=CARTESIAN_POINT('Ctrl Pts',(0.900002971484041,1.2238959908032,0.641061424759933));
#13796=CARTESIAN_POINT('Ctrl Pts',(0.900002662567364,1.22064256379503,0.648296551655426));
#13797=CARTESIAN_POINT('Ctrl Pts',(0.900001146653719,1.21656554418039,0.655104870690721));
#13798=CARTESIAN_POINT('Ctrl Pts',(0.900000540233788,1.21172928299109,0.66132323772617));
#13799=CARTESIAN_POINT('Ctrl Pts',(0.900000424918953,1.21080963534652,0.66250570210793));
#13800=CARTESIAN_POINT('Ctrl Pts',(0.900000351402035,1.20986240082127,0.663666762843393));
#13801=CARTESIAN_POINT('Ctrl Pts',(0.900000346234225,1.20888784277449,0.664805176146358));
#13802=CARTESIAN_POINT('Ctrl Pts',(0.900000336405833,1.20703438079614,0.666970266034709));
#13803=CARTESIAN_POINT('Ctrl Pts',(0.900000571869483,1.20508211779724,0.669053482241208));
#13804=CARTESIAN_POINT('Ctrl Pts',(0.900000903580486,1.20303784749416,0.671051418948595));
#13805=CARTESIAN_POINT('Ctrl Pts',(0.900001825932764,1.19735357006848,0.676606861644505));
#13806=CARTESIAN_POINT('Ctrl Pts',(0.900003332967427,1.19102482074992,0.681443262092019));
#13807=CARTESIAN_POINT('Ctrl Pts',(0.900003895332687,1.18421635668109,0.685507797106414));
#13808=CARTESIAN_POINT('Ctrl Pts',(0.900004254598985,1.17986677848026,0.688104419886002));
#13809=CARTESIAN_POINT('Ctrl Pts',(0.9000042929279,1.17532044218795,0.69038534615497));
#13810=CARTESIAN_POINT('Ctrl Pts',(0.900003997675654,1.17061445353731,0.692327416690341));
#13811=CARTESIAN_POINT('Ctrl Pts',(0.900003537640084,1.16328200409216,0.695353376818313));
#13812=CARTESIAN_POINT('Ctrl Pts',(0.900002259964378,1.15564663185935,0.697524398440697));
#13813=CARTESIAN_POINT('Ctrl Pts',(0.900001215101098,1.14785635641255,0.698771715080855));
#13814=CARTESIAN_POINT('Ctrl Pts',(0.900000537649455,1.14280542295857,0.699580430175527));
#13815=CARTESIAN_POINT('Ctrl Pts',(0.899999997568109,1.13768876957788,0.699999998835552));
#13816=CARTESIAN_POINT('Ctrl Pts',(0.899999999937205,1.13254484130906,0.7));
#13817=CARTESIAN_POINT('Ctrl Pts',(0.9,1.266106713614,0.));
#13818=CARTESIAN_POINT('Ctrl Pts',(0.9,1.26053025554556,0.100869097599589));
#13819=CARTESIAN_POINT('Ctrl Pts',(0.9,1.25495230648558,0.201739398169819));
#13820=CARTESIAN_POINT('Ctrl Pts',(0.9,1.24378819189631,0.403576374532447));
#13821=CARTESIAN_POINT('Ctrl Pts',(0.9,1.23820188085298,0.504545629805417));
#13822=CARTESIAN_POINT('Ctrl Pts',(0.9,1.23261418131727,0.605513513251856));
#13823=CARTESIAN_POINT('Ctrl Pts',(0.900000000000002,-1.266106713614,-8.15320033709099E-17));
#13824=CARTESIAN_POINT('Ctrl Pts',(0.908871090277923,-1.25552568177643,
0.201930159665972));
#13825=CARTESIAN_POINT('Ctrl Pts',(0.917742329685194,-1.24494466498547,
0.403860313587921));
#13826=CARTESIAN_POINT('Ctrl Pts',(0.926613720860141,-1.23436366359623,
0.605790461668883));
#13827=CARTESIAN_POINT('Ctrl Pts',(0.697441255022372,-1.25280938151844,
-5.71013218131409E-5));
#13828=CARTESIAN_POINT('Ctrl Pts',(0.706712389899261,-1.24222855501813,
0.201872952723963));
#13829=CARTESIAN_POINT('Ctrl Pts',(0.71598368260269,-1.23164774534186,0.403803000441224));
#13830=CARTESIAN_POINT('Ctrl Pts',(0.725255135891715,-1.22106695288555,
0.605733041729342));
#13831=CARTESIAN_POINT('Ctrl Pts',(0.494899146035781,-1.23832021354117,
-0.000119230777047918));
#13832=CARTESIAN_POINT('Ctrl Pts',(0.504570354086872,-1.2277396148863,0.201810708652083));
#13833=CARTESIAN_POINT('Ctrl Pts',(0.514241728780064,-1.21715903502506,
0.403740641123913));
#13834=CARTESIAN_POINT('Ctrl Pts',(0.523913273026478,-1.20657847439907,
0.605670566527588));
#13835=CARTESIAN_POINT('Ctrl Pts',(0.292373353339556,-1.22258574808743,
-0.000186633859775947));
#13836=CARTESIAN_POINT('Ctrl Pts',(0.302444661323169,-1.21200540195431,
0.201743181663441));
#13837=CARTESIAN_POINT('Ctrl Pts',(0.312516144861689,-1.20142507679253,
0.403672989556125));
#13838=CARTESIAN_POINT('Ctrl Pts',(0.322587807049886,-1.190844773096,0.605602789690272));
#13839=CARTESIAN_POINT('',(0.32407846024449,-1.19096124572524,0.605603291426262));
#13840=CARTESIAN_POINT('Ctrl Pts',(0.292382661757373,-1.22257596919059,
-1.26634813746307E-16));
#13841=CARTESIAN_POINT('Ctrl Pts',(0.302948004341657,-1.21203750712027,
0.201867748891544));
#13842=CARTESIAN_POINT('Ctrl Pts',(0.313513270922098,-1.20149926476964,
0.403735512620674));
#13843=CARTESIAN_POINT('Ctrl Pts',(0.324078460244491,-1.19096124572524,
0.605603291426262));
#13844=CARTESIAN_POINT('Ctrl Pts',(0.324078460244487,-1.19096124572524,
0.605603291426262));
#13845=CARTESIAN_POINT('Ctrl Pts',(0.515976798438381,-1.20595780001216,
0.605571001180369));
#13846=CARTESIAN_POINT('Ctrl Pts',(0.707956283694857,-1.21982772882273,
0.605541108414459));
#13847=CARTESIAN_POINT('Ctrl Pts',(0.900000000000001,-1.23261418131727,
0.605513513251856));
#13848=CARTESIAN_POINT('Ctrl Pts',(0.906632491847682,-1.13298681949577,
0.7));
#13849=CARTESIAN_POINT('Ctrl Pts',(0.714963137593258,-1.12022681655782,
0.7));
#13850=CARTESIAN_POINT('Ctrl Pts',(0.52336552158394,-1.10638609587519,0.7));
#13851=CARTESIAN_POINT('Ctrl Pts',(0.331856371369197,-1.09142177001972,
0.7));
#13852=CARTESIAN_POINT('Ctrl Pts',(0.904714827274509,-1.16179226195561,
0.7));
#13853=CARTESIAN_POINT('Ctrl Pts',(0.712937153454425,-1.14901967286075,
0.69999980360337));
#13854=CARTESIAN_POINT('Ctrl Pts',(0.521230340369869,-1.13516557394852,
0.700000229443053));
#13855=CARTESIAN_POINT('Ctrl Pts',(0.329608751265076,-1.12018616744754,
0.7));
#13856=CARTESIAN_POINT('Ctrl Pts',(0.901389714107723,-1.21173913866089,
0.676722045797292));
#13857=CARTESIAN_POINT('Ctrl Pts',(0.709425477581998,-1.19894546296063,
0.676731074746188));
#13858=CARTESIAN_POINT('Ctrl Pts',(0.517526696841433,-1.18506766126723,
0.67674067107047));
#13859=CARTESIAN_POINT('Ctrl Pts',(0.325711429829026,-1.17006296935233,
0.676751229163451));
#13860=CARTESIAN_POINT('Ctrl Pts',(0.900079298017777,-1.23142303740181,
0.627132481749528));
#13861=CARTESIAN_POINT('Ctrl Pts',(0.708040181852795,-1.21863106773591,
0.627155851652593));
#13862=CARTESIAN_POINT('Ctrl Pts',(0.516066269599777,-1.20475540724405,
0.627181012790208));
#13863=CARTESIAN_POINT('Ctrl Pts',(0.324172915772929,-1.18975243096407,
0.627208352638976));
#13864=CARTESIAN_POINT('Ctrl Pts',(0.900000000000001,-1.23261418131727,
0.605513513251856));
#13865=CARTESIAN_POINT('Ctrl Pts',(0.707956283694857,-1.21982772882273,
0.605541108414459));
#13866=CARTESIAN_POINT('Ctrl Pts',(0.515976798438381,-1.20595780001216,
0.605571001180369));
#13867=CARTESIAN_POINT('Ctrl Pts',(0.324078460244487,-1.19096124572524,
0.605603291426262));
#13868=CARTESIAN_POINT('',(0.3318563713692,-1.09142177001972,0.7));
#13869=CARTESIAN_POINT('Origin',(0.3318563713692,-1.09142177001972,0.6));
#13870=CARTESIAN_POINT('Ctrl Pts',(0.899999999937167,-1.13254484130906,
0.7));
#13871=CARTESIAN_POINT('Ctrl Pts',(0.710543123935439,-1.11990737114256,
0.7));
#13872=CARTESIAN_POINT('Ctrl Pts',(0.521156529292483,-1.10621348751457,
0.7));
#13873=CARTESIAN_POINT('Ctrl Pts',(0.331856371369197,-1.09142177001972,
0.7));
#13874=CARTESIAN_POINT('Origin',(5.4,-8.11656130105013E-18,0.7));
#13875=CARTESIAN_POINT('',(0.3318563713692,1.09142177001972,0.7));
#13876=CARTESIAN_POINT('',(0.3318563713692,-0.7,0.7));
#13877=CARTESIAN_POINT('Ctrl Pts',(0.3318563713692,1.09142177001972,0.7));
#13878=CARTESIAN_POINT('Ctrl Pts',(0.521156529292483,1.10621348751457,0.7));
#13879=CARTESIAN_POINT('Ctrl Pts',(0.710543123935438,1.11990737114256,0.7));
#13880=CARTESIAN_POINT('Ctrl Pts',(0.899999999937165,1.13254484130906,0.7));
#13881=CARTESIAN_POINT('Ctrl Pts',(0.292373353339556,1.22258574808743,-0.000186633859776018));
#13882=CARTESIAN_POINT('Ctrl Pts',(0.30244466132317,1.21200540195431,0.20174318166344));
#13883=CARTESIAN_POINT('Ctrl Pts',(0.31251614486169,1.20142507679253,0.403672989556124));
#13884=CARTESIAN_POINT('Ctrl Pts',(0.322587807049886,1.190844773096,0.605602789690271));
#13885=CARTESIAN_POINT('Ctrl Pts',(0.494899146035781,1.23832021354117,-0.000119230777047989));
#13886=CARTESIAN_POINT('Ctrl Pts',(0.504570354086872,1.2277396148863,0.201810708652083));
#13887=CARTESIAN_POINT('Ctrl Pts',(0.514241728780064,1.21715903502506,0.403740641123914));
#13888=CARTESIAN_POINT('Ctrl Pts',(0.523913273026478,1.20657847439907,0.605670566527587));
#13889=CARTESIAN_POINT('Ctrl Pts',(0.697441255022371,1.25280938151844,-5.71013218130602E-5));
#13890=CARTESIAN_POINT('Ctrl Pts',(0.70671238989926,1.24222855501813,0.201872952723963));
#13891=CARTESIAN_POINT('Ctrl Pts',(0.715983682602689,1.23164774534186,0.403803000441224));
#13892=CARTESIAN_POINT('Ctrl Pts',(0.725255135891714,1.22106695288555,0.605733041729342));
#13893=CARTESIAN_POINT('Ctrl Pts',(0.9,1.266106713614,1.73472347597681E-18));
#13894=CARTESIAN_POINT('Ctrl Pts',(0.908871090277921,1.25552568177643,0.201930159665973));
#13895=CARTESIAN_POINT('Ctrl Pts',(0.917742329685192,1.24494466498547,0.403860313587921));
#13896=CARTESIAN_POINT('Ctrl Pts',(0.92661372086014,1.23436366359623,0.605790461668883));
#13897=CARTESIAN_POINT('',(0.32407846024449,1.19096124572524,0.605603291426262));
#13898=CARTESIAN_POINT('Ctrl Pts',(0.9,1.23261418131727,0.605513513251856));
#13899=CARTESIAN_POINT('Ctrl Pts',(0.707956283694857,1.21982772882273,0.605541108414459));
#13900=CARTESIAN_POINT('Ctrl Pts',(0.515976798438382,1.20595780001216,0.60557100118037));
#13901=CARTESIAN_POINT('Ctrl Pts',(0.32407846024449,1.19096124572524,0.605603291426262));
#13902=CARTESIAN_POINT('Ctrl Pts',(0.324078460244491,1.19096124572524,0.605603291426262));
#13903=CARTESIAN_POINT('Ctrl Pts',(0.313513270922098,1.20149926476964,0.403735512620674));
#13904=CARTESIAN_POINT('Ctrl Pts',(0.302948004341658,1.21203750712026,0.201867748891544));
#13905=CARTESIAN_POINT('Ctrl Pts',(0.292382661757373,1.22257596919059,3.4477629085039E-17));
#13906=CARTESIAN_POINT('Ctrl Pts',(0.3318563713692,1.09142177001972,0.7));
#13907=CARTESIAN_POINT('Ctrl Pts',(0.523365521583941,1.10638609587519,0.7));
#13908=CARTESIAN_POINT('Ctrl Pts',(0.714963137593258,1.12022681655782,0.7));
#13909=CARTESIAN_POINT('Ctrl Pts',(0.906632491847681,1.13298681949577,0.7));
#13910=CARTESIAN_POINT('Ctrl Pts',(0.329608751265078,1.12018616744754,0.7));
#13911=CARTESIAN_POINT('Ctrl Pts',(0.52123034036987,1.13516557394852,0.700000229443053));
#13912=CARTESIAN_POINT('Ctrl Pts',(0.712937153454426,1.14901967286075,0.699999803603371));
#13913=CARTESIAN_POINT('Ctrl Pts',(0.904714827274509,1.16179226195561,0.700000000000001));
#13914=CARTESIAN_POINT('Ctrl Pts',(0.325711429829028,1.17006296935233,0.676751229163452));
#13915=CARTESIAN_POINT('Ctrl Pts',(0.517526696841433,1.18506766126723,0.67674067107047));
#13916=CARTESIAN_POINT('Ctrl Pts',(0.709425477581997,1.19894546296063,0.676731074746189));
#13917=CARTESIAN_POINT('Ctrl Pts',(0.901389714107722,1.21173913866089,0.676722045797292));
#13918=CARTESIAN_POINT('Ctrl Pts',(0.324172915772932,1.18975243096407,0.627208352638976));
#13919=CARTESIAN_POINT('Ctrl Pts',(0.516066269599778,1.20475540724405,0.627181012790208));
#13920=CARTESIAN_POINT('Ctrl Pts',(0.708040181852794,1.21863106773591,0.627155851652593));
#13921=CARTESIAN_POINT('Ctrl Pts',(0.900079298017776,1.23142303740181,0.627132481749528));
#13922=CARTESIAN_POINT('Ctrl Pts',(0.32407846024449,1.19096124572524,0.605603291426262));
#13923=CARTESIAN_POINT('Ctrl Pts',(0.515976798438382,1.20595780001216,0.60557100118037));
#13924=CARTESIAN_POINT('Ctrl Pts',(0.707956283694857,1.21982772882273,0.605541108414459));
#13925=CARTESIAN_POINT('Ctrl Pts',(0.9,1.23261418131727,0.605513513251856));
#13926=CARTESIAN_POINT('Origin',(0.331856371369202,1.09142177001972,0.6));
#13927=CARTESIAN_POINT('Origin',(0.331856371369202,1.09142177001972,0.6));
#13928=CARTESIAN_POINT('Origin',(0.331856371369201,1.09142177001972,0.6));
#13929=CARTESIAN_POINT('Origin',(0.331856371369202,1.09142177001972,0.6));
#13930=CARTESIAN_POINT('Origin',(10.4681436286308,1.08420482079361,0.6));
#13931=CARTESIAN_POINT('Origin',(10.4681436276939,1.08420482084454,0.6));
#13932=CARTESIAN_POINT('',(10.5680065821063,1.08420482079361,0.605233595624295));
#13933=CARTESIAN_POINT('Origin',(10.4681436286308,1.08420482079361,0.6));
#13934=CARTESIAN_POINT('Origin',(10.4681436286308,1.08420482079361,0.6));
#13935=CARTESIAN_POINT('Origin',(0.3318563713692,-1.09142177001972,0.6));
#13936=CARTESIAN_POINT('Origin',(0.331856371369201,-1.09142177001972,0.6));
#13937=CARTESIAN_POINT('Origin',(0.3318563713692,-1.09142177001972,0.6));
#13938=CARTESIAN_POINT('Origin',(0.3318563713692,-0.7,0.6));
#13939=CARTESIAN_POINT('Ctrl Pts',(0.2922895713475,-1.22266882276207,-0.00177864096060679));
#13940=CARTESIAN_POINT('Ctrl Pts',(0.302885944515497,-1.21209940820877,
0.200681988163859));
#13941=CARTESIAN_POINT('Ctrl Pts',(0.313482241236256,-1.20153021465708,
0.403142632212487));
#13942=CARTESIAN_POINT('Ctrl Pts',(0.324078460244491,-1.19096124572524,
0.605603291426262));
#13943=CARTESIAN_POINT('Ctrl Pts',(0.264022491930188,-1.22039553779506,
-0.000415890128406236));
#13944=CARTESIAN_POINT('Ctrl Pts',(0.274621881512248,-1.20982222712748,
0.202044379074236));
#13945=CARTESIAN_POINT('Ctrl Pts',(0.285221154833576,-1.19924944554801,
0.404504681968985));
#13946=CARTESIAN_POINT('Ctrl Pts',(0.29582042516239,-1.18867654001483,0.606964977361795));
#13947=CARTESIAN_POINT('Ctrl Pts',(0.216712469170969,-1.1940874043406,0.000690255297866666));
#13948=CARTESIAN_POINT('Ctrl Pts',(0.227319688237882,-1.18351239299796,
0.203150045648192));
#13949=CARTESIAN_POINT('Ctrl Pts',(0.237926932441998,-1.17293746916702,
0.405609838636422));
#13950=CARTESIAN_POINT('Ctrl Pts',(0.248534117816369,-1.1623628476683,0.608069650238703));
#13951=CARTESIAN_POINT('Ctrl Pts',(0.200219987929043,-1.14439035743082,
-0.00103956457010847));
#13952=CARTESIAN_POINT('Ctrl Pts',(0.210830491339948,-1.13382006821851,
0.201420337884579));
#13953=CARTESIAN_POINT('Ctrl Pts',(0.221440906577676,-1.12324995278282,
0.403880253819325));
#13954=CARTESIAN_POINT('Ctrl Pts',(0.232051411471599,-1.11268010558856,
0.606340179010355));
#13955=CARTESIAN_POINT('Ctrl Pts',(0.200161975173303,-1.12312592850316,
-0.00214651389202307));
#13956=CARTESIAN_POINT('Ctrl Pts',(0.210772455448684,-1.11255764422181,
0.200313510564959));
#13957=CARTESIAN_POINT('Ctrl Pts',(0.221382936352032,-1.1019895901204,0.402773547004277));
#13958=CARTESIAN_POINT('Ctrl Pts',(0.231993417893744,-1.09142177001972,
0.605233595624295));
#13959=CARTESIAN_POINT('Origin',(10.4681436286308,-1.08420482109828,0.6));
#13960=CARTESIAN_POINT('',(10.5680065821063,-1.08420482079361,0.605233595624295));
#13961=CARTESIAN_POINT('Origin',(10.4681436286308,-1.08420482099672,0.600000000000001));
#13962=CARTESIAN_POINT('Origin',(10.4681436286308,-1.08420482109828,0.6));
#13963=CARTESIAN_POINT('Origin',(10.4681436286308,0.7,0.6));
#13964=CARTESIAN_POINT('',(10.5680065821063,0.7,0.605233595624295));
#13965=CARTESIAN_POINT('Ctrl Pts',(10.599839982685,-1.11594741464673,-0.00218387205330164));
#13966=CARTESIAN_POINT('Ctrl Pts',(10.5892288496247,-1.10536637943871,0.200288608282177));
#13967=CARTESIAN_POINT('Ctrl Pts',(10.5786177161011,-1.0947855138519,0.402761097457634));
#13968=CARTESIAN_POINT('Ctrl Pts',(10.5680065821063,-1.08420482079362,0.605233595624295));
#13969=CARTESIAN_POINT('Ctrl Pts',(10.5997613205547,-1.14474784499259,-0.000682909193257743));
#13970=CARTESIAN_POINT('Ctrl Pts',(10.5891501209488,-1.13416481604349,0.201789447273867));
#13971=CARTESIAN_POINT('Ctrl Pts',(10.5785391399155,-1.12358205581644,0.404261829287571));
#13972=CARTESIAN_POINT('Ctrl Pts',(10.5679279386544,-1.11299934606825,0.606734202078189));
#13973=CARTESIAN_POINT('Ctrl Pts',(10.5764119435127,-1.19466846760808,0.000702210001053139));
#13974=CARTESIAN_POINT('Ctrl Pts',(10.5658041809617,-1.18408222297768,0.203174550667819));
#13975=CARTESIAN_POINT('Ctrl Pts',(10.5551963844732,-1.17349608774572,0.405646894856767));
#13976=CARTESIAN_POINT('Ctrl Pts',(10.544588659013,-1.16291012508165,0.608119251464957));
#13977=CARTESIAN_POINT('Ctrl Pts',(10.5269342003857,-1.21442651155969,-0.000858270497959616));
#13978=CARTESIAN_POINT('Ctrl Pts',(10.5163317654776,-1.20384274018949,0.201614467507756));
#13979=CARTESIAN_POINT('Ctrl Pts',(10.5057293269973,-1.1932591813998,0.404087216090532));
#13980=CARTESIAN_POINT('Ctrl Pts',(10.4951269905998,-1.18267571840064,0.606559974437339));
#13981=CARTESIAN_POINT('Ctrl Pts',(10.5053655128635,-1.21565094114741,-0.0019246498908503));
#13982=CARTESIAN_POINT('Ctrl Pts',(10.4947646468921,-1.20506932615592,0.200548282383137));
#13983=CARTESIAN_POINT('Ctrl Pts',(10.4841638390504,-1.19448787589602,0.403021225840181));
#13984=CARTESIAN_POINT('Ctrl Pts',(10.4735630903435,-1.18390659316268,0.605494180667945));
#13985=CARTESIAN_POINT('Ctrl Pts',(10.5997255308004,-1.11583328740478,1.02782365951626E-16));
#13986=CARTESIAN_POINT('Ctrl Pts',(10.589152548365,-1.10529029582828,0.201744523047832));
#13987=CARTESIAN_POINT('Ctrl Pts',(10.5785795654695,-1.09474747266587,0.40348905487273));
#13988=CARTESIAN_POINT('Ctrl Pts',(10.5680065821063,-1.08420482079362,0.605233595624295));
#13989=CARTESIAN_POINT('Ctrl Pts',(10.5053638082297,1.21564923960921,-0.0018920919656423));
#13990=CARTESIAN_POINT('Ctrl Pts',(10.4947635104759,1.20506819181477,0.200569987667808));
#13991=CARTESIAN_POINT('Ctrl Pts',(10.4841632708454,1.19448730873444,0.403032078483127));
#13992=CARTESIAN_POINT('Ctrl Pts',(10.4735630903435,1.18390659316268,0.605494180667945));
#13993=CARTESIAN_POINT('Ctrl Pts',(10.5341220579192,1.21401666636749,-0.000470252816738081));
#13994=CARTESIAN_POINT('Ctrl Pts',(10.5235196325477,1.20343268662274,0.201991562854702));
#13995=CARTESIAN_POINT('Ctrl Pts',(10.5129172908767,1.19284910679518,0.404453403808947));
#13996=CARTESIAN_POINT('Ctrl Pts',(10.5023149573519,1.18226542681329,0.606915239027137));
#13997=CARTESIAN_POINT('Ctrl Pts',(10.5827170203615,1.18801090922716,0.000717463067903341));
#13998=CARTESIAN_POINT('Ctrl Pts',(10.5721088691741,1.17742555398174,0.203178921531494));
#13999=CARTESIAN_POINT('Ctrl Pts',(10.5615007184277,1.16684027916303,0.405640383775807));
#14000=CARTESIAN_POINT('Ctrl Pts',(10.5508925935528,1.15625520969485,0.60810185787831));
#14001=CARTESIAN_POINT('Ctrl Pts',(10.5997792798033,1.13754603572512,-0.00102559206997387));
#14002=CARTESIAN_POINT('Ctrl Pts',(10.5891686973038,1.12696411138589,0.201435946515793));
#14003=CARTESIAN_POINT('Ctrl Pts',(10.5785581831385,1.11638231376635,0.40389749513889));
#14004=CARTESIAN_POINT('Ctrl Pts',(10.5679475995174,1.10580071474959,0.606359050464716));
#14005=CARTESIAN_POINT('Ctrl Pts',(10.5998382764002,1.11594571320176,-0.00215131420076595));
#14006=CARTESIAN_POINT('Ctrl Pts',(10.5892277121014,1.10536524516024,0.200310313518148));
#14007=CARTESIAN_POINT('Ctrl Pts',(10.5786171473394,1.09478494672192,0.402771950076102));
#14008=CARTESIAN_POINT('Ctrl Pts',(10.5680065821063,1.08420482079361,0.605233595624295));
#14009=CARTESIAN_POINT('Ctrl Pts',(10.5680065821063,1.08420482079361,0.605233595624295));
#14010=CARTESIAN_POINT('Ctrl Pts',(10.5785795654695,1.09474747266587,0.40348905487273));
#14011=CARTESIAN_POINT('Ctrl Pts',(10.589152548365,1.10529029582828,0.201744523047831));
#14012=CARTESIAN_POINT('Ctrl Pts',(10.5997255308004,1.11583328740478,1.07661275727811E-16));
#14013=CARTESIAN_POINT('Ctrl Pts',(10.1947388861048,1.09885088260187,0.7));
#14014=CARTESIAN_POINT('Ctrl Pts',(10.285877616441,1.09404209584202,0.7));
#14015=CARTESIAN_POINT('Ctrl Pts',(10.3770124662346,1.0891584122264,0.7));
#14016=CARTESIAN_POINT('Ctrl Pts',(10.4681436286308,1.08420482079361,0.7));
#14017=CARTESIAN_POINT('Ctrl Pts',(10.196260416419,1.12768774893097,0.700000000000001));
#14018=CARTESIAN_POINT('Ctrl Pts',(10.2874149314686,1.12287675076168,0.699999949550842));
#14019=CARTESIAN_POINT('Ctrl Pts',(10.3785648662465,1.11799094453753,0.700000051218742));
#14020=CARTESIAN_POINT('Ctrl Pts',(10.4697107510168,1.11303515260326,0.7));
#14021=CARTESIAN_POINT('Ctrl Pts',(10.1988975981852,1.17766904563614,0.67669140632491));
#14022=CARTESIAN_POINT('Ctrl Pts',(10.2900793016129,1.17285439035486,0.676693724638983));
#14023=CARTESIAN_POINT('Ctrl Pts',(10.3812557252598,1.16796482352885,0.676696026813929));
#14024=CARTESIAN_POINT('Ctrl Pts',(10.4724269697127,1.16300539549315,0.676698381019544));
#14025=CARTESIAN_POINT('Ctrl Pts',(10.1999375452555,1.19737868557977,0.627098033786781));
#14026=CARTESIAN_POINT('Ctrl Pts',(10.2911301919381,1.19256517083271,0.627104033151799));
#14027=CARTESIAN_POINT('Ctrl Pts',(10.382317043787,1.18767684023183,0.627110048826767));
#14028=CARTESIAN_POINT('Ctrl Pts',(10.4734985149421,1.18271860027509,0.627116141711795));
#14029=CARTESIAN_POINT('Ctrl Pts',(10.1999999975038,1.19856231440453,0.605472757505366));
#14030=CARTESIAN_POINT('Ctrl Pts',(10.2911933328565,1.19375025772558,0.605479840815741));
#14031=CARTESIAN_POINT('Ctrl Pts',(10.3823809652617,1.18886335120032,0.605486986548286));
#14032=CARTESIAN_POINT('Ctrl Pts',(10.4735630903435,1.18390659316268,0.605494180667944));
#14033=CARTESIAN_POINT('Ctrl Pts',(0.200159601751749,1.12312829248604,-0.00219180147311912));
#14034=CARTESIAN_POINT('Ctrl Pts',(0.210770873167554,1.11255922017607,0.200283318842441));
#14035=CARTESIAN_POINT('Ctrl Pts',(0.221382145211419,1.10199037808008,0.402758451142111));
#14036=CARTESIAN_POINT('Ctrl Pts',(0.231993417893744,1.09142177001972,0.605233595624295));
#14037=CARTESIAN_POINT('Ctrl Pts',(0.200236952094631,1.15148086499205,-0.000715869007730825));
#14038=CARTESIAN_POINT('Ctrl Pts',(0.210848310847714,1.14090905181173,0.201759082033021));
#14039=CARTESIAN_POINT('Ctrl Pts',(0.221459381762758,1.13033759660317,0.404234066901971));
#14040=CARTESIAN_POINT('Ctrl Pts',(0.232070742664217,1.11976621744484,0.606709040139042));
#14041=CARTESIAN_POINT('Ctrl Pts',(0.222806696702742,1.20067708175657,0.000669311976984441));
#14042=CARTESIAN_POINT('Ctrl Pts',(0.233413416075889,1.19010082554658,0.203144236955742));
#14043=CARTESIAN_POINT('Ctrl Pts',(0.244020198555212,1.17952469009474,0.405619164345205));
#14044=CARTESIAN_POINT('Ctrl Pts',(0.254626870458834,1.16894881850735,0.608094110943904));
#14045=CARTESIAN_POINT('Ctrl Pts',(0.271086891015657,1.22096622390789,-0.000801865493577694));
#14046=CARTESIAN_POINT('Ctrl Pts',(0.281686280594249,1.21039315447922,0.201673594461172));
#14047=CARTESIAN_POINT('Ctrl Pts',(0.292285672737775,1.1998203699977,0.404149068703718));
#14048=CARTESIAN_POINT('Ctrl Pts',(0.302884933932915,1.18924771644243,0.606624555877912));
#14049=CARTESIAN_POINT('Ctrl Pts',(0.292287201081515,1.22267118699778,-0.00182392867695869));
#14050=CARTESIAN_POINT('Ctrl Pts',(0.302884364349574,1.21210098433295,0.200651796350731));
#14051=CARTESIAN_POINT('Ctrl Pts',(0.313481451159089,1.20153100270242,0.403127536304793));
#14052=CARTESIAN_POINT('Ctrl Pts',(0.324078460244491,1.19096124572524,0.605603291426262));
#14053=CARTESIAN_POINT('Origin',(10.6002740930491,1.4,-0.0104671912485891));
#14054=CARTESIAN_POINT('Origin',(0.331856371369202,1.09142177001972,0.6));
#14055=CARTESIAN_POINT('',(0.3318563713692,1.09142177001972,0.9));
#14056=CARTESIAN_POINT('',(0.0322675109428288,1.09142177001972,0.615700786872883));
#14057=CARTESIAN_POINT('Origin',(0.3318563713692,1.09142177001972,0.6));
#14058=CARTESIAN_POINT('',(0.308522637995069,1.39004019713626,0.616809874278785));
#14059=CARTESIAN_POINT('Origin',(0.331856371369202,1.09142177001972,0.6));
#14060=CARTESIAN_POINT('Origin',(0.331856371369201,1.09142177001972,0.6));
#14061=CARTESIAN_POINT('Origin',(10.4681436286308,1.08420482079361,0.6));
#14062=CARTESIAN_POINT('',(10.4681436286308,1.08420482109828,0.9));
#14063=CARTESIAN_POINT('',(10.4844020137689,1.3833101379008,0.616482542003833));
#14064=CARTESIAN_POINT('Origin',(10.4681436258201,1.08420482094639,0.6));
#14065=CARTESIAN_POINT('',(10.7677324890572,1.08420482079361,0.615700786872884));
#14066=CARTESIAN_POINT('Origin',(10.4681436286308,1.08420482079361,0.6));
#14067=CARTESIAN_POINT('Origin',(10.4681436286308,1.08420482079362,0.6));
#14068=CARTESIAN_POINT('Origin',(0.3318563713692,-1.09142177001972,0.6));
#14069=CARTESIAN_POINT('',(0.3318563713692,-1.09142177001972,0.9));
#14070=CARTESIAN_POINT('',(0.308522637995069,-1.39004019713626,0.616809874278785));
#14071=CARTESIAN_POINT('Origin',(0.3318563713692,-1.09142177001972,0.6));
#14072=CARTESIAN_POINT('',(0.0322675109428289,-1.09142177001972,0.615700786872884));
#14073=CARTESIAN_POINT('Origin',(0.3318563713692,-1.09142177001972,0.6));
#14074=CARTESIAN_POINT('Origin',(0.331856371369201,-1.09142177001972,0.6));
#14075=CARTESIAN_POINT('Origin',(0.3318563713692,-0.7,0.6));
#14076=CARTESIAN_POINT('',(0.0322675109428288,-0.7,0.615700786872883));
#14077=CARTESIAN_POINT('',(0.3318563713692,-0.7,0.9));
#14078=CARTESIAN_POINT('Ctrl Pts',(0.276048389810261,-1.42252533450788,
-0.00533608639730399));
#14079=CARTESIAN_POINT('Ctrl Pts',(0.28687338241706,-1.4116967417008,0.202045878554724));
#14080=CARTESIAN_POINT('Ctrl Pts',(0.297698133178874,-1.40086836142621,
0.409427865329919));
#14081=CARTESIAN_POINT('Ctrl Pts',(0.308522637995069,-1.39004019713626,
0.616809874278785));
#14082=CARTESIAN_POINT('Ctrl Pts',(0.191246496057484,-1.41570630783033,
-0.00124775669238285));
#14083=CARTESIAN_POINT('Ctrl Pts',(0.202080757839133,-1.40486573978029,
0.206133102090467));
#14084=CARTESIAN_POINT('Ctrl Pts',(0.212914648880055,-1.39402634701096,
0.413514041581016));
#14085=CARTESIAN_POINT('Ctrl Pts',(0.223748532748767,-1.38318608000504,
0.620894932085382));
#14086=CARTESIAN_POINT('Ctrl Pts',(0.0492682973509243,-1.33685850703924,
0.00207719607616587));
#14087=CARTESIAN_POINT('Ctrl Pts',(0.0601266125734448,-1.32601270457081,
0.209456583216085));
#14088=CARTESIAN_POINT('Ctrl Pts',(0.0709850253737815,-1.3151666447344,
0.416835949794532));
#14089=CARTESIAN_POINT('Ctrl Pts',(0.0818432319483421,-1.30432109509162,
0.624215353109623));
#14090=CARTESIAN_POINT('Ctrl Pts',(-0.000163444061205068,-1.18769013309795,
-0.00311869847265479));
#14091=CARTESIAN_POINT('Ctrl Pts',(0.0107049555364969,-1.17685886333949,
0.204261034729081));
#14092=CARTESIAN_POINT('Ctrl Pts',(0.0215730900970294,-1.16602762920277,
0.411640782964944));
#14093=CARTESIAN_POINT('Ctrl Pts',(0.0324414916763936,-1.15519677672624,
0.619020537031064));
#14094=CARTESIAN_POINT('Ctrl Pts',(-0.00033748371827097,-1.12389640457412,
-0.0064395729582146));
#14095=CARTESIAN_POINT('Ctrl Pts',(0.0105308471731094,-1.11307128361434,
0.200940534347673));
#14096=CARTESIAN_POINT('Ctrl Pts',(0.0213991787230862,-1.10224640406117,
0.408320654220332));
#14097=CARTESIAN_POINT('Ctrl Pts',(0.0322675109428289,-1.09142177001972,
0.615700786872884));
#14098=CARTESIAN_POINT('Ctrl Pts',(0.27632692456468,-1.42224670711126,5.13911829758129E-17));
#14099=CARTESIAN_POINT('Ctrl Pts',(0.287059068122268,-1.41151099373342,
0.20560326985903));
#14100=CARTESIAN_POINT('Ctrl Pts',(0.297790973931072,-1.40077548928706,
0.411206561171438));
#14101=CARTESIAN_POINT('Ctrl Pts',(0.308522637995069,-1.39004019713626,
0.616809874278785));
#14102=CARTESIAN_POINT('Ctrl Pts',(0.0322675109428289,-1.09142177001972,
0.615700786872884));
#14103=CARTESIAN_POINT('Ctrl Pts',(0.0215116733095221,-1.10213436178043,
0.410467178800746));
#14104=CARTESIAN_POINT('Ctrl Pts',(0.0107558363321879,-1.11284719399673,
0.205233583245308));
#14105=CARTESIAN_POINT('Ctrl Pts',(1.76901136968166E-16,-1.12356026268968,
-7.45931094670027E-17));
#14106=CARTESIAN_POINT('Origin',(10.4681436286308,-1.08420482109828,0.6));
#14107=CARTESIAN_POINT('',(10.7677324890572,-1.08420482079361,0.615700786872884));
#14108=CARTESIAN_POINT('',(10.4844020137689,-1.3833101379008,0.616482542003833));
#14109=CARTESIAN_POINT('Origin',(10.4681436286308,-1.08420482079361,0.600000000000001));
#14110=CARTESIAN_POINT('',(10.4681436258201,-1.08420482094639,0.9));
#14111=CARTESIAN_POINT('Origin',(10.4681436286308,-1.08420482109828,0.6));
#14112=CARTESIAN_POINT('Origin',(10.4681436286308,-1.08420482079361,0.6));
#14113=CARTESIAN_POINT('Origin',(10.4681436286308,0.7,0.6));
#14114=CARTESIAN_POINT('',(10.7677324890572,0.7,0.615700786872884));
#14115=CARTESIAN_POINT('',(10.4681436286308,0.7,0.9));
#14116=CARTESIAN_POINT('Ctrl Pts',(10.4681436286308,-1.08420482079361,0.9));
#14117=CARTESIAN_POINT('Ctrl Pts',(9.02115959826777,-1.16285813221549,0.9));
#14118=CARTESIAN_POINT('Ctrl Pts',(5.64262097844114,-1.30550334054488,0.9));
#14119=CARTESIAN_POINT('Ctrl Pts',(2.25816172369615,-1.24194126716656,0.9));
#14120=CARTESIAN_POINT('Ctrl Pts',(0.331856371369198,-1.09142177001972,
0.9));
#14121=CARTESIAN_POINT('Ctrl Pts',(10.4728449957889,-1.17069581622255,0.9));
#14122=CARTESIAN_POINT('Ctrl Pts',(9.02515960257209,-1.24945398332951,0.900002463983243));
#14123=CARTESIAN_POINT('Ctrl Pts',(5.64406008560805,-1.39235654229312,0.899995181674544));
#14124=CARTESIAN_POINT('Ctrl Pts',(2.25481214769604,-1.3286896492945,0.900006992415263));
#14125=CARTESIAN_POINT('Ctrl Pts',(0.325113511056834,-1.17771496230318,
0.9));
#14126=CARTESIAN_POINT('Ctrl Pts',(10.4809942371438,-1.32061731204901,0.830050158657121));
#14127=CARTESIAN_POINT('Ctrl Pts',(9.03210079995546,-1.3995487214628,0.829938185878055));
#14128=CARTESIAN_POINT('Ctrl Pts',(5.64656962219688,-1.54290142969263,0.82970437227026));
#14129=CARTESIAN_POINT('Ctrl Pts',(2.24896854757963,-1.47903552984056,0.829838703712927));
#14130=CARTESIAN_POINT('Ctrl Pts',(0.313425270489114,-1.32729771265557,
0.830156825336737));
#14131=CARTESIAN_POINT('Ctrl Pts',(10.4842082875648,-1.37974615923803,0.681348425135383));
#14132=CARTESIAN_POINT('Ctrl Pts',(9.03482793853036,-1.45862084618981,0.681058092399338));
#14133=CARTESIAN_POINT('Ctrl Pts',(5.64753778607331,-1.60187726023264,0.68045297450285));
#14134=CARTESIAN_POINT('Ctrl Pts',(2.24670449952385,-1.53809938127555,0.680799765935021));
#14135=CARTESIAN_POINT('Ctrl Pts',(0.308806004580392,-1.38641375285276,
0.681625057916928));
#14136=CARTESIAN_POINT('Ctrl Pts',(10.4844020137689,-1.3833101379008,0.616482542003833));
#14137=CARTESIAN_POINT('Ctrl Pts',(9.03499042108131,-1.46211428773623,0.616139856494792));
#14138=CARTESIAN_POINT('Ctrl Pts',(5.64759185703765,-1.60522711936681,0.615422163720642));
#14139=CARTESIAN_POINT('Ctrl Pts',(2.24657199659733,-1.54153220865049,0.615835494619844));
#14140=CARTESIAN_POINT('Ctrl Pts',(0.308522637995066,-1.39004019713626,
0.616809874278785));
#14141=CARTESIAN_POINT('Ctrl Pts',(0.308522637995066,-1.39004019713626,
0.616809874278785));
#14142=CARTESIAN_POINT('Ctrl Pts',(2.24657199659733,-1.54153220865049,0.615835494619844));
#14143=CARTESIAN_POINT('Ctrl Pts',(5.64759185703765,-1.60522711936681,0.615422163720642));
#14144=CARTESIAN_POINT('Ctrl Pts',(9.03499042108131,-1.46211428773623,0.616139856494792));
#14145=CARTESIAN_POINT('Ctrl Pts',(10.4844020137689,-1.3833101379008,0.616482542003833));
#14146=CARTESIAN_POINT('Ctrl Pts',(10.4681436258201,-1.08420482094639,0.900000000000001));
#14147=CARTESIAN_POINT('Ctrl Pts',(9.02115959639274,-1.16285813229465,0.9));
#14148=CARTESIAN_POINT('Ctrl Pts',(5.64262097750198,-1.30550334052724,0.9));
#14149=CARTESIAN_POINT('Ctrl Pts',(2.25816172369615,-1.24194126716656,0.9));
#14150=CARTESIAN_POINT('Ctrl Pts',(0.331856371369198,-1.09142177001972,
0.9));
#14151=CARTESIAN_POINT('Ctrl Pts',(10.8003433549902,-1.11672267507076,-0.00655160349952438));
#14152=CARTESIAN_POINT('Ctrl Pts',(10.7894730668347,-1.10588321133639,0.200865850630566));
#14153=CARTESIAN_POINT('Ctrl Pts',(10.7786027781932,-1.09504392553578,0.408283314033857));
#14154=CARTESIAN_POINT('Ctrl Pts',(10.7677324890572,-1.08420482079361,0.615700786872885));
#14155=CARTESIAN_POINT('Ctrl Pts',(10.8001073672393,-1.20312439623403,-0.00204868896805508));
#14156=CARTESIAN_POINT('Ctrl Pts',(10.7892368724076,-1.19227880391739,0.205368384315645));
#14157=CARTESIAN_POINT('Ctrl Pts',(10.7783670568079,-1.18143370221047,0.41278551899075));
#14158=CARTESIAN_POINT('Ctrl Pts',(10.7674965587017,-1.17058839661753,0.620202606234566));
#14159=CARTESIAN_POINT('Ctrl Pts',(10.7300137544668,-1.35289768637741,0.00210488808650419));
#14160=CARTESIAN_POINT('Ctrl Pts',(10.7191538066016,-1.34204221082848,0.209521911971666));
#14161=CARTESIAN_POINT('Ctrl Pts',(10.7082938463195,-1.33118673671862,0.416938933985702));
#14162=CARTESIAN_POINT('Ctrl Pts',(10.6974340169938,-1.32033143065575,0.624355970618915));
#14163=CARTESIAN_POINT('Ctrl Pts',(10.5816241002662,-1.4121605627967,-0.00257485550010117));
#14164=CARTESIAN_POINT('Ctrl Pts',(10.5707805459565,-1.4013126969686,0.204843391064434));
#14165=CARTESIAN_POINT('Ctrl Pts',(10.5599369567012,-1.39046512672587,0.412261650129749));
#14166=CARTESIAN_POINT('Ctrl Pts',(10.5490937145378,-1.37961751361469,0.619679923312015));
#14167=CARTESIAN_POINT('Ctrl Pts',(10.5169176890673,-1.41583338198674,-0.00577403633861717));
#14168=CARTESIAN_POINT('Ctrl Pts',(10.5060789456421,-1.40499213715574,0.201644806368331));
#14169=CARTESIAN_POINT('Ctrl Pts',(10.4952403861233,-1.39415105487295,0.40906366572247));
#14170=CARTESIAN_POINT('Ctrl Pts',(10.4844020137689,-1.3833101379008,0.616482542003833));
#14171=CARTESIAN_POINT('Ctrl Pts',(10.8,-1.11638029377732,-2.51534904016637E-17));
#14172=CARTESIAN_POINT('Ctrl Pts',(10.7892441634977,-1.10565496086826,0.205233586491178));
#14173=CARTESIAN_POINT('Ctrl Pts',(10.7784883265195,-1.09492980219801,0.410467182062988));
#14174=CARTESIAN_POINT('Ctrl Pts',(10.7677324890572,-1.08420482079361,0.615700786872885));
#14175=CARTESIAN_POINT('Ctrl Pts',(10.4844020137689,-1.3833101379008,0.616482542003833));
#14176=CARTESIAN_POINT('Ctrl Pts',(10.4951398148107,-1.39405045994841,0.410988344812119));
#14177=CARTESIAN_POINT('Ctrl Pts',(10.5058777995597,-1.40479094425298,0.205494164234945));
#14178=CARTESIAN_POINT('Ctrl Pts',(10.5166159648474,-1.4155315881283,-2.5652223401007E-16));
#14179=CARTESIAN_POINT('Ctrl Pts',(10.5169125872774,1.41582827901939,-0.0056764044152427));
#14180=CARTESIAN_POINT('Ctrl Pts',(10.5060755445066,1.40498873522851,0.20170989432247));
#14181=CARTESIAN_POINT('Ctrl Pts',(10.4952386855848,1.39414935393528,0.409096209702196));
#14182=CARTESIAN_POINT('Ctrl Pts',(10.4844020137689,1.3833101379008,0.616482542003833));
#14183=CARTESIAN_POINT('Ctrl Pts',(10.6031877991504,1.41093118264609,-0.00141083033817288));
#14184=CARTESIAN_POINT('Ctrl Pts',(10.5923442181457,1.40008262840665,0.205974657203891));
#14185=CARTESIAN_POINT('Ctrl Pts',(10.5815009048179,1.38923496752292,0.413360205434192));
#14186=CARTESIAN_POINT('Ctrl Pts',(10.5706576147941,1.37838663885266,0.62074571708141));
#14187=CARTESIAN_POINT('Ctrl Pts',(10.7489822201969,1.33286898269122,0.00215046584238339));
#14188=CARTESIAN_POINT('Ctrl Pts',(10.7381210493968,1.32201618867047,0.209534855263179));
#14189=CARTESIAN_POINT('Ctrl Pts',(10.7272598662103,1.31116338896628,0.416919242515175));
#14190=CARTESIAN_POINT('Ctrl Pts',(10.716398780155,1.30031077634578,0.624303643734563));
#14191=CARTESIAN_POINT('Ctrl Pts',(10.8001612475457,1.18151886169146,-0.00307678645922502));
#14192=CARTESIAN_POINT('Ctrl Pts',(10.7892926103682,1.17067663552019,0.20430785074418));
#14193=CARTESIAN_POINT('Ctrl Pts',(10.7784241800195,1.15983442267521,0.41169249890798));
#14194=CARTESIAN_POINT('Ctrl Pts',(10.7675555412906,1.14899250266155,0.619077151394146));
#14195=CARTESIAN_POINT('Ctrl Pts',(10.8003382383521,1.11671757294177,-0.00645397222975308));
#14196=CARTESIAN_POINT('Ctrl Pts',(10.7894696557425,1.1058798099729,0.200930938146656));
#14197=CARTESIAN_POINT('Ctrl Pts',(10.778601072647,1.09504222488243,0.408315857793383));
#14198=CARTESIAN_POINT('Ctrl Pts',(10.7677324890572,1.08420482079361,0.615700786872884));
#14199=CARTESIAN_POINT('Ctrl Pts',(10.5166159648474,1.4155315881283,3.37837396946483E-16));
#14200=CARTESIAN_POINT('Ctrl Pts',(10.5058777995597,1.40479094425298,0.205494164234944));
#14201=CARTESIAN_POINT('Ctrl Pts',(10.4951398148107,1.39405045994841,0.41098834481212));
#14202=CARTESIAN_POINT('Ctrl Pts',(10.4844020137689,1.3833101379008,0.616482542003833));
#14203=CARTESIAN_POINT('Ctrl Pts',(10.7677324890572,1.08420482079361,0.615700786872884));
#14204=CARTESIAN_POINT('Ctrl Pts',(10.7784883265195,1.09492980219801,0.410467182062988));
#14205=CARTESIAN_POINT('Ctrl Pts',(10.7892441634977,1.10565496086826,0.205233586491177));
#14206=CARTESIAN_POINT('Ctrl Pts',(10.8,1.11638029377732,-4.7271214720368E-17));
#14207=CARTESIAN_POINT('Ctrl Pts',(0.3318563713692,1.09142177001972,0.9));
#14208=CARTESIAN_POINT('Ctrl Pts',(1.77658538561441,1.20431139287985,0.9));
#14209=CARTESIAN_POINT('Ctrl Pts',(5.15852145577913,1.31798734362749,0.900000000000001));
#14210=CARTESIAN_POINT('Ctrl Pts',(8.53883158814675,1.18907590268945,0.9));
#14211=CARTESIAN_POINT('Ctrl Pts',(10.4681436286308,1.08420482079361,0.9));
#14212=CARTESIAN_POINT('Ctrl Pts',(0.325113511056836,1.17771496230318,0.9));
#14213=CARTESIAN_POINT('Ctrl Pts',(1.77238748853623,1.29094597754667,0.900005244311447));
#14214=CARTESIAN_POINT('Ctrl Pts',(5.15940689953628,1.40489117512763,0.899995532233175));
#14215=CARTESIAN_POINT('Ctrl Pts',(8.54259780483314,1.2757067056985,0.90000328531099));
#14216=CARTESIAN_POINT('Ctrl Pts',(10.4728449957889,1.17069581622255,0.9));
#14217=CARTESIAN_POINT('Ctrl Pts',(0.313425270489116,1.32729771265557,0.830156825336737));
#14218=CARTESIAN_POINT('Ctrl Pts',(1.76508272830699,1.44110107554431,0.829918234118879));
#14219=CARTESIAN_POINT('Ctrl Pts',(5.16095094050242,1.55552201031752,0.829677185710002));
#14220=CARTESIAN_POINT('Ctrl Pts',(8.54913632089268,1.4258591912674,0.829900861618366));
#14221=CARTESIAN_POINT('Ctrl Pts',(10.4809942371438,1.32061731204901,0.830050158657121));
#14222=CARTESIAN_POINT('Ctrl Pts',(0.308806004580394,1.38641375285276,0.681625057916928));
#14223=CARTESIAN_POINT('Ctrl Pts',(1.76222987578798,1.50017797416985,0.681006088930498));
#14224=CARTESIAN_POINT('Ctrl Pts',(5.16154986224672,1.61450132085358,0.68038246417749));
#14225=CARTESIAN_POINT('Ctrl Pts',(8.55170115551887,1.48491240850707,0.680961314820656));
#14226=CARTESIAN_POINT('Ctrl Pts',(10.4842082875648,1.37974615923803,0.681348425135383));
#14227=CARTESIAN_POINT('Ctrl Pts',(0.308522637995068,1.39004019713626,0.616809874278785));
#14228=CARTESIAN_POINT('Ctrl Pts',(1.76205965694675,1.50365920577193,0.616079089534579));
#14229=CARTESIAN_POINT('Ctrl Pts',(5.16158497046229,1.61783515152865,0.615338844765104));
#14230=CARTESIAN_POINT('Ctrl Pts',(8.55185322351876,1.48838233768137,0.616025627991778));
#14231=CARTESIAN_POINT('Ctrl Pts',(10.4844020137689,1.3833101379008,0.616482542003833));
#14232=CARTESIAN_POINT('Ctrl Pts',(10.4844020137689,1.3833101379008,0.616482542003833));
#14233=CARTESIAN_POINT('Ctrl Pts',(8.55185322351876,1.48838233768137,0.616025627991778));
#14234=CARTESIAN_POINT('Ctrl Pts',(5.16158497046229,1.61783515152865,0.615338844765104));
#14235=CARTESIAN_POINT('Ctrl Pts',(1.76205965694675,1.50365920577193,0.616079089534579));
#14236=CARTESIAN_POINT('Ctrl Pts',(0.308522637995068,1.39004019713626,0.616809874278785));
#14237=CARTESIAN_POINT('Ctrl Pts',(0.3318563713692,1.09142177001972,0.9));
#14238=CARTESIAN_POINT('Ctrl Pts',(1.77658538561441,1.20431139287985,0.9));
#14239=CARTESIAN_POINT('Ctrl Pts',(5.15852145577913,1.31798734362749,0.900000000000001));
#14240=CARTESIAN_POINT('Ctrl Pts',(8.53883158814675,1.18907590268945,0.9));
#14241=CARTESIAN_POINT('Ctrl Pts',(10.4681436286308,1.08420482079361,0.9));
#14242=CARTESIAN_POINT('Ctrl Pts',(-0.000344602063817145,1.12390349461883,
-0.00657539908256866));
#14243=CARTESIAN_POINT('Ctrl Pts',(0.0105261016091243,1.11307601020539,
0.200849983592616));
#14244=CARTESIAN_POINT('Ctrl Pts',(0.0213968059409475,1.10224876730309,
0.408275378840013));
#14245=CARTESIAN_POINT('Ctrl Pts',(0.0322675109428289,1.09142177001972,
0.615700786872884));
#14246=CARTESIAN_POINT('Ctrl Pts',(-0.000112549170678945,1.2089618047365,
-0.00214756610981592));
#14247=CARTESIAN_POINT('Ctrl Pts',(0.0107584275574203,1.19812589474889,
0.205277296000037));
#14248=CARTESIAN_POINT('Ctrl Pts',(0.021628504370896,1.18729063034778,0.412702239156743));
#14249=CARTESIAN_POINT('Ctrl Pts',(0.0324994852542487,1.17645511229507,
0.620127120417125));
#14250=CARTESIAN_POINT('Ctrl Pts',(0.0675181008536004,1.35659180908255,
0.00201426213057289));
#14251=CARTESIAN_POINT('Ctrl Pts',(0.0783748317004002,1.34574224493831,
0.20943904356877));
#14252=CARTESIAN_POINT('Ctrl Pts',(0.0892318011706237,1.33489254525337,
0.416863803530356));
#14253=CARTESIAN_POINT('Ctrl Pts',(0.100088380073201,1.32404321751407,0.624288602298589));
#14254=CARTESIAN_POINT('Ctrl Pts',(0.212439875011655,1.41741816253371,-0.00240566592686199));
#14255=CARTESIAN_POINT('Ctrl Pts',(0.223274062163905,1.40657840226088,0.20502076110302));
#14256=CARTESIAN_POINT('Ctrl Pts',(0.234108278795672,1.39573903465802,0.412447205628077));
#14257=CARTESIAN_POINT('Ctrl Pts',(0.244942059060342,1.38489960928785,0.619873667633733));
#14258=CARTESIAN_POINT('Ctrl Pts',(0.276041299849618,1.42253242682652,-0.00547191373834488));
#14259=CARTESIAN_POINT('Ctrl Pts',(0.286868655882245,1.41170146982041,0.201955326984501));
#14260=CARTESIAN_POINT('Ctrl Pts',(0.297695769965166,1.40087072543886,0.409382589539965));
#14261=CARTESIAN_POINT('Ctrl Pts',(0.308522637995069,1.39004019713626,0.616809874278785));
#14262=CARTESIAN_POINT('Ctrl Pts',(2.26869304592592E-17,1.12356026268968,
-3.16587034365767E-17));
#14263=CARTESIAN_POINT('Ctrl Pts',(0.0107558363321878,1.11284719399672,
0.205233583245308));
#14264=CARTESIAN_POINT('Ctrl Pts',(0.0215116733095221,1.10213436178043,
0.410467178800746));
#14265=CARTESIAN_POINT('Ctrl Pts',(0.0322675109428289,1.09142177001972,
0.615700786872884));
#14266=CARTESIAN_POINT('Ctrl Pts',(0.308522637995069,1.39004019713626,0.616809874278785));
#14267=CARTESIAN_POINT('Ctrl Pts',(0.297790973931072,1.40077548928706,0.411206561171438));
#14268=CARTESIAN_POINT('Ctrl Pts',(0.287059068122271,1.41151099373341,0.205603269859031));
#14269=CARTESIAN_POINT('Ctrl Pts',(0.276326924564681,1.42224670711126,-2.68882138776405E-16));
#14270=CARTESIAN_POINT('Ctrl Pts',(10.5166159648474,-1.4155315881283,0.));
#14271=CARTESIAN_POINT('Ctrl Pts',(10.5064062201588,-1.40475637621136,0.205603291426271));
#14272=CARTESIAN_POINT('Ctrl Pts',(10.4961964754701,-1.39398116429443,0.411206582852543));
#14273=CARTESIAN_POINT('Ctrl Pts',(10.4859867307814,-1.38320595237749,0.616809874278814));
#14274=CARTESIAN_POINT('Ctrl Pts',(7.10318628475318,-1.599994843061,0.));
#14275=CARTESIAN_POINT('Ctrl Pts',(7.09978773046573,-1.58921963114407,0.205603291426271));
#14276=CARTESIAN_POINT('Ctrl Pts',(7.09638917617828,-1.57844441922713,0.411206582852543));
#14277=CARTESIAN_POINT('Ctrl Pts',(7.09299062189083,-1.5676692073102,0.616809874278814));
#14278=CARTESIAN_POINT('Ctrl Pts',(3.68975660465893,-1.68747752195839,0.));
#14279=CARTESIAN_POINT('Ctrl Pts',(3.69316924077269,-1.67670231004145,0.205603291426272));
#14280=CARTESIAN_POINT('Ctrl Pts',(3.69658187688646,-1.66592709812452,0.411206582852543));
#14281=CARTESIAN_POINT('Ctrl Pts',(3.69999451300023,-1.65515188620758,0.616809874278814));
#14282=CARTESIAN_POINT('Ctrl Pts',(0.276326924564679,-1.42224670711126,
0.));
#14283=CARTESIAN_POINT('Ctrl Pts',(0.286550751079662,-1.41147149519433,
0.205603291426271));
#14284=CARTESIAN_POINT('Ctrl Pts',(0.296774577594646,-1.40069628327739,
0.411206582852543));
#14285=CARTESIAN_POINT('Ctrl Pts',(0.306998404109629,-1.38992107136046,
0.616809874278814));
#14286=CARTESIAN_POINT('Origin',(0.,-1.4,0.));
#14287=CARTESIAN_POINT('Origin',(5.4,-8.13935059369636E-18,0.9));
#14288=CARTESIAN_POINT('Ctrl Pts',(0.276326924564679,1.42224670711126,0.));
#14289=CARTESIAN_POINT('Ctrl Pts',(0.286550751079662,1.41147149519433,0.205603291426271));
#14290=CARTESIAN_POINT('Ctrl Pts',(0.296774577594645,1.40069628327739,0.411206582852543));
#14291=CARTESIAN_POINT('Ctrl Pts',(0.306998404109628,1.38992107136046,0.616809874278814));
#14292=CARTESIAN_POINT('Ctrl Pts',(3.68975660465893,1.68747752195839,0.));
#14293=CARTESIAN_POINT('Ctrl Pts',(3.6931692407727,1.67670231004145,0.205603291426271));
#14294=CARTESIAN_POINT('Ctrl Pts',(3.69658187688646,1.66592709812452,0.411206582852543));
#14295=CARTESIAN_POINT('Ctrl Pts',(3.69999451300023,1.65515188620758,0.616809874278814));
#14296=CARTESIAN_POINT('Ctrl Pts',(7.10318628475318,1.599994843061,0.));
#14297=CARTESIAN_POINT('Ctrl Pts',(7.09978773046573,1.58921963114407,0.205603291426271));
#14298=CARTESIAN_POINT('Ctrl Pts',(7.09638917617828,1.57844441922713,0.411206582852543));
#14299=CARTESIAN_POINT('Ctrl Pts',(7.09299062189083,1.5676692073102,0.616809874278814));
#14300=CARTESIAN_POINT('Ctrl Pts',(10.5166159648474,1.4155315881283,0.));
#14301=CARTESIAN_POINT('Ctrl Pts',(10.5064062201588,1.40475637621136,0.205603291426271));
#14302=CARTESIAN_POINT('Ctrl Pts',(10.4961964754701,1.39398116429443,0.411206582852543));
#14303=CARTESIAN_POINT('Ctrl Pts',(10.4859867307814,1.38320595237749,0.616809874278814));
#14304=CARTESIAN_POINT('Origin',(10.8,1.4,0.));
#22111=UNCERTAINTY_MEASURE_WITH_UNIT(LENGTH_MEASURE(0.001),#22130,
'DISTANCE_ACCURACY_VALUE',
'Maximum model space distance between geometric entities at asserted c
onnectivities');
#22117=UNCERTAINTY_MEASURE_WITH_UNIT(LENGTH_MEASURE(0.001),#22130,
'DISTANCE_ACCURACY_VALUE',
'Maximum model space distance between geometric entities at asserted c
onnectivities');
#22123=(
GEOMETRIC_REPRESENTATION_CONTEXT(3)
GLOBAL_UNCERTAINTY_ASSIGNED_CONTEXT((#22111))
GLOBAL_UNIT_ASSIGNED_CONTEXT((#22130,#22132,#22133))
REPRESENTATION_CONTEXT('','3D')
);
#22129=(
GEOMETRIC_REPRESENTATION_CONTEXT(3)
GLOBAL_UNCERTAINTY_ASSIGNED_CONTEXT((#22117))
GLOBAL_UNIT_ASSIGNED_CONTEXT((#22130,#22132,#22133))
REPRESENTATION_CONTEXT('','3D')
);
#22130=(
LENGTH_UNIT()
NAMED_UNIT(*)
SI_UNIT(.CENTI.,.METRE.)
);
#22132=(
NAMED_UNIT(*)
PLANE_ANGLE_UNIT()
SI_UNIT($,.RADIAN.)
);
#22133=(
NAMED_UNIT(*)
SI_UNIT($,.STERADIAN.)
SOLID_ANGLE_UNIT()
);
#22139=SHAPE_DEFINITION_REPRESENTATION(#22150,#22177);
#22150=PRODUCT_DEFINITION_SHAPE('',$,#22189);
#22177=SHAPE_REPRESENTATION('',(#9088),#22123);
#22183=PRODUCT_DEFINITION_CONTEXT('part definition',#22218,'design');
#22189=PRODUCT_DEFINITION('2026-11-10-05-10-49-232',
'Upper structural shell',#22200,#22183);
#22200=PRODUCT_DEFINITION_FORMATION('',$,#22225);
#22218=APPLICATION_CONTEXT(
'Core Data for Automotive Mechanical Design Process');
#22219=PRODUCT_CONTEXT('part definition',#22218,'mechanical');
#22225=PRODUCT('2026-11-10-05-10-49-232','Upper structural shell',$,(#22219));
#22235=PRESENTATION_STYLE_ASSIGNMENT((#22243));
#22243=SURFACE_STYLE_USAGE(.BOTH.,#22251);
#22251=SURFACE_SIDE_STYLE('',(#22259));
#22259=SURFACE_STYLE_FILL_AREA(#22267);
#22267=FILL_AREA_STYLE('Structural dark blue',(#22275));
#22275=FILL_AREA_STYLE_COLOUR('Structural dark blue',#22283);
#22283=COLOUR_RGB('Structural dark blue',0.0901960784313725,0.270588235294118,
0.513725490196078);
ENDSEC;
END-ISO-10303-21;
